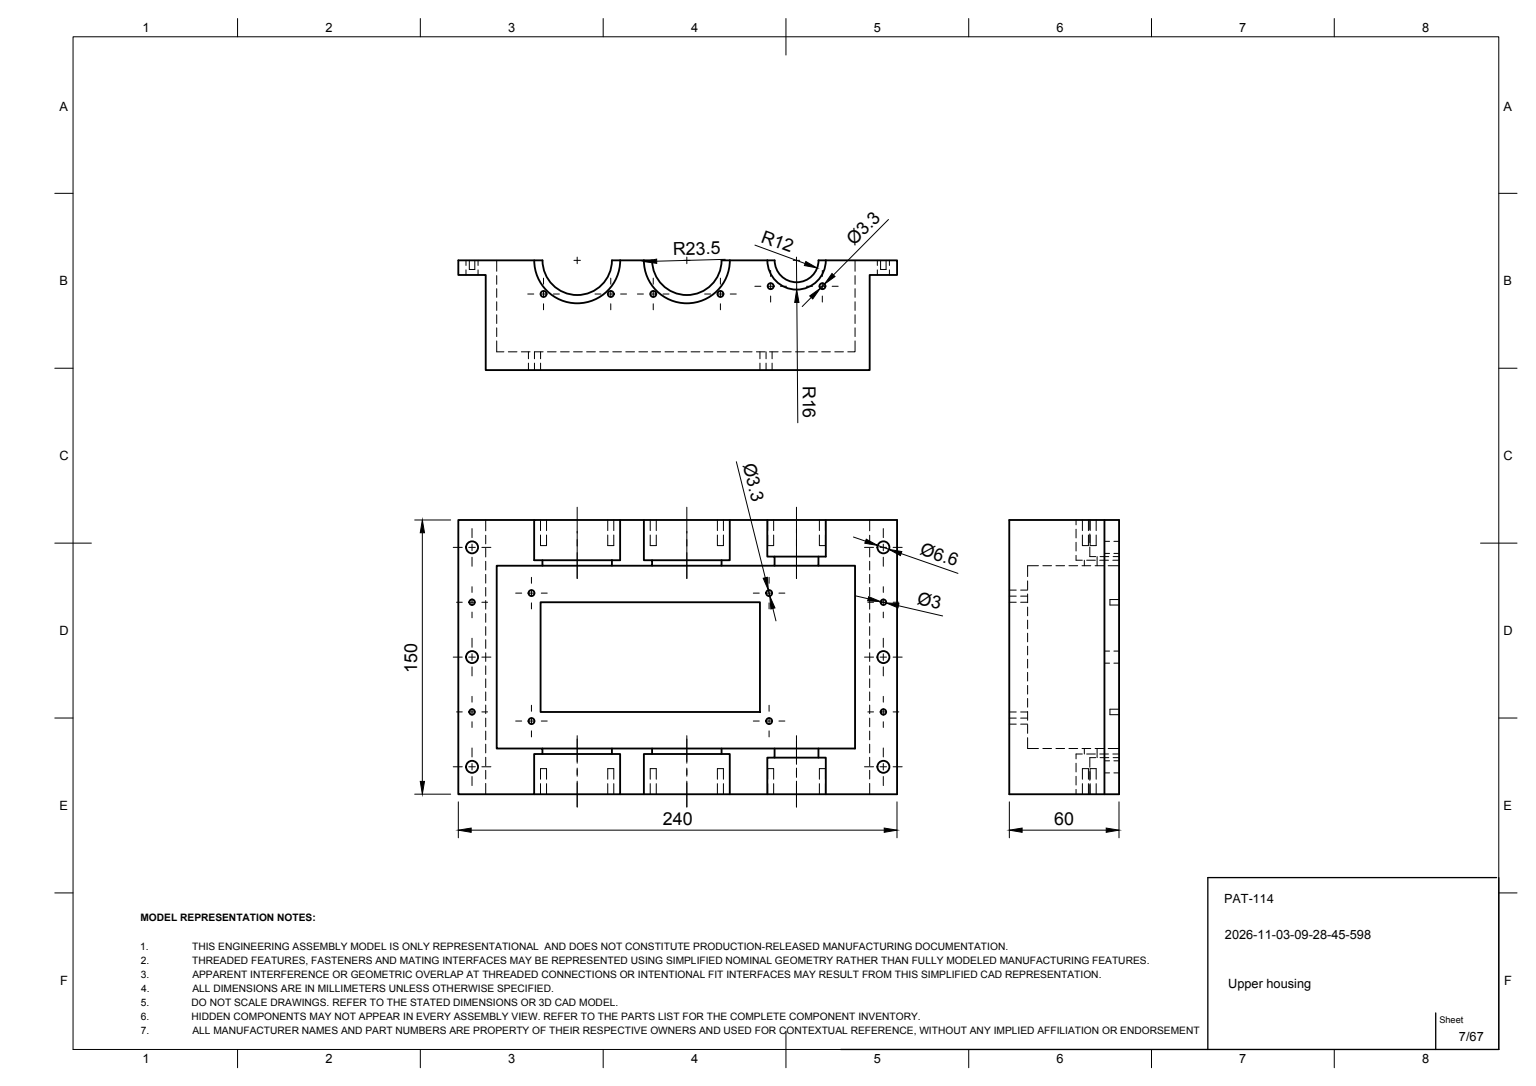
ISO-10303-21;
HEADER;
/* Generated by software containing ST-Developer
 * from STEP Tools, Inc. (www.steptools.com) 
 */

FILE_DESCRIPTION(
/* description */ ('Two-stage gear reducer in split housing'),
/* implementation_level */ '2;1');

FILE_NAME(
/* name */ 'Upper housing.step',
/* time_stamp */ '2026-10-28T03:22:31-07:00',
/* author */ (''),
/* organization */ (''),
/* preprocessor_version */ 'ST-DEVELOPER v20.2',
/* originating_system */ 'Autodesk Translation Framework v15.17.0.0',
/* authorisation */ '');

FILE_SCHEMA (('AUTOMOTIVE_DESIGN { 1 0 10303 214 3 1 1 }'));
ENDSEC;

DATA;
#10=MECHANICAL_DESIGN_GEOMETRIC_PRESENTATION_REPRESENTATION('',(#1236),#73366);
#1124=SHAPE_REPRESENTATION_RELATIONSHIP('SRR','None',#73611,#1180);
#1180=ADVANCED_BREP_SHAPE_REPRESENTATION('',(#1307),#73307);
#1236=STYLED_ITEM('',(#73967),#1307);
#1307=MANIFOLD_SOLID_BREP('Body1',#16124);
#1422=FACE_BOUND('',#3081,.T.);
#1423=FACE_BOUND('',#3082,.T.);
#1424=FACE_BOUND('',#3083,.T.);
#1425=FACE_BOUND('',#3084,.T.);
#1426=FACE_BOUND('',#3085,.T.);
#1427=FACE_BOUND('',#3089,.T.);
#1428=FACE_BOUND('',#3090,.T.);
#1429=FACE_BOUND('',#3091,.T.);
#1430=FACE_BOUND('',#3092,.T.);
#1431=FACE_BOUND('',#3093,.T.);
#1432=FACE_BOUND('',#3094,.T.);
#1433=FACE_BOUND('',#3097,.T.);
#1434=FACE_BOUND('',#3098,.T.);
#1435=FACE_BOUND('',#3099,.T.);
#1436=FACE_BOUND('',#3100,.T.);
#1437=FACE_BOUND('',#3101,.T.);
#1438=FACE_BOUND('',#3102,.T.);
#1439=FACE_BOUND('',#3138,.T.);
#1440=FACE_BOUND('',#3139,.T.);
#1441=FACE_BOUND('',#3140,.T.);
#1442=FACE_BOUND('',#3141,.T.);
#1443=FACE_BOUND('',#3142,.T.);
#1444=FACE_BOUND('',#3159,.T.);
#1445=FACE_BOUND('',#3160,.T.);
#1446=FACE_BOUND('',#3161,.T.);
#1447=FACE_BOUND('',#3164,.T.);
#1448=FACE_BOUND('',#3165,.T.);
#1449=FACE_BOUND('',#3166,.T.);
#1450=FACE_BOUND('',#3171,.T.);
#1451=FACE_BOUND('',#3172,.T.);
#1452=FACE_BOUND('',#3173,.T.);
#1453=FACE_BOUND('',#3174,.T.);
#1454=FACE_BOUND('',#3175,.T.);
#1455=FACE_BOUND('',#3178,.T.);
#1456=FACE_BOUND('',#3179,.T.);
#1457=FACE_BOUND('',#3180,.T.);
#1458=FACE_BOUND('',#3181,.T.);
#1459=FACE_BOUND('',#3182,.T.);
#1654=PLANE('',#17019);
#1655=PLANE('',#17020);
#1656=PLANE('',#17021);
#1657=PLANE('',#17022);
#1658=PLANE('',#17026);
#1659=PLANE('',#17030);
#1660=PLANE('',#17034);
#1661=PLANE('',#17038);
#1662=PLANE('',#17039);
#1663=PLANE('',#17046);
#1664=PLANE('',#17055);
#1665=PLANE('',#17057);
#1666=PLANE('',#17066);
#1667=PLANE('',#17073);
#1668=PLANE('',#17076);
#1669=PLANE('',#17077);
#1670=PLANE('',#17080);
#1671=PLANE('',#17083);
#1672=PLANE('',#17086);
#1673=PLANE('',#17089);
#1674=PLANE('',#17090);
#1675=PLANE('',#17098);
#1676=PLANE('',#17101);
#1677=PLANE('',#17102);
#1678=PLANE('',#17105);
#1679=PLANE('',#17108);
#1680=PLANE('',#17111);
#1681=PLANE('',#17114);
#1682=PLANE('',#17117);
#1683=PLANE('',#17121);
#1684=PLANE('',#17126);
#1685=PLANE('',#17127);
#1686=PLANE('',#17135);
#1687=PLANE('',#17138);
#1688=PLANE('',#17141);
#1689=PLANE('',#17144);
#1690=PLANE('',#17157);
#1691=PLANE('',#17158);
#1692=PLANE('',#17159);
#1693=PLANE('',#17160);
#1694=PLANE('',#17161);
#1695=PLANE('',#17162);
#1696=PLANE('',#17163);
#1697=PLANE('',#17164);
#1698=PLANE('',#17165);
#1699=PLANE('',#17166);
#2100=FACE_OUTER_BOUND('',#3061,.T.);
#2101=FACE_OUTER_BOUND('',#3062,.T.);
#2102=FACE_OUTER_BOUND('',#3063,.T.);
#2103=FACE_OUTER_BOUND('',#3064,.T.);
#2104=FACE_OUTER_BOUND('',#3065,.T.);
#2105=FACE_OUTER_BOUND('',#3066,.T.);
#2106=FACE_OUTER_BOUND('',#3067,.T.);
#2107=FACE_OUTER_BOUND('',#3068,.T.);
#2108=FACE_OUTER_BOUND('',#3069,.T.);
#2109=FACE_OUTER_BOUND('',#3070,.T.);
#2110=FACE_OUTER_BOUND('',#3071,.T.);
#2111=FACE_OUTER_BOUND('',#3072,.T.);
#2112=FACE_OUTER_BOUND('',#3073,.T.);
#2113=FACE_OUTER_BOUND('',#3074,.T.);
#2114=FACE_OUTER_BOUND('',#3075,.T.);
#2115=FACE_OUTER_BOUND('',#3076,.T.);
#2116=FACE_OUTER_BOUND('',#3077,.T.);
#2117=FACE_OUTER_BOUND('',#3078,.T.);
#2118=FACE_OUTER_BOUND('',#3079,.T.);
#2119=FACE_OUTER_BOUND('',#3080,.T.);
#2120=FACE_OUTER_BOUND('',#3086,.T.);
#2121=FACE_OUTER_BOUND('',#3087,.T.);
#2122=FACE_OUTER_BOUND('',#3088,.T.);
#2123=FACE_OUTER_BOUND('',#3095,.T.);
#2124=FACE_OUTER_BOUND('',#3096,.T.);
#2125=FACE_OUTER_BOUND('',#3103,.T.);
#2126=FACE_OUTER_BOUND('',#3104,.T.);
#2127=FACE_OUTER_BOUND('',#3105,.T.);
#2128=FACE_OUTER_BOUND('',#3106,.T.);
#2129=FACE_OUTER_BOUND('',#3107,.T.);
#2130=FACE_OUTER_BOUND('',#3108,.T.);
#2131=FACE_OUTER_BOUND('',#3109,.T.);
#2132=FACE_OUTER_BOUND('',#3110,.T.);
#2133=FACE_OUTER_BOUND('',#3111,.T.);
#2134=FACE_OUTER_BOUND('',#3112,.T.);
#2135=FACE_OUTER_BOUND('',#3113,.T.);
#2136=FACE_OUTER_BOUND('',#3114,.T.);
#2137=FACE_OUTER_BOUND('',#3115,.T.);
#2138=FACE_OUTER_BOUND('',#3116,.T.);
#2139=FACE_OUTER_BOUND('',#3117,.T.);
#2140=FACE_OUTER_BOUND('',#3118,.T.);
#2141=FACE_OUTER_BOUND('',#3119,.T.);
#2142=FACE_OUTER_BOUND('',#3120,.T.);
#2143=FACE_OUTER_BOUND('',#3121,.T.);
#2144=FACE_OUTER_BOUND('',#3122,.T.);
#2145=FACE_OUTER_BOUND('',#3123,.T.);
#2146=FACE_OUTER_BOUND('',#3124,.T.);
#2147=FACE_OUTER_BOUND('',#3125,.T.);
#2148=FACE_OUTER_BOUND('',#3126,.T.);
#2149=FACE_OUTER_BOUND('',#3127,.T.);
#2150=FACE_OUTER_BOUND('',#3128,.T.);
#2151=FACE_OUTER_BOUND('',#3129,.T.);
#2152=FACE_OUTER_BOUND('',#3130,.T.);
#2153=FACE_OUTER_BOUND('',#3131,.T.);
#2154=FACE_OUTER_BOUND('',#3132,.T.);
#2155=FACE_OUTER_BOUND('',#3133,.T.);
#2156=FACE_OUTER_BOUND('',#3134,.T.);
#2157=FACE_OUTER_BOUND('',#3135,.T.);
#2158=FACE_OUTER_BOUND('',#3136,.T.);
#2159=FACE_OUTER_BOUND('',#3137,.T.);
#2160=FACE_OUTER_BOUND('',#3143,.T.);
#2161=FACE_OUTER_BOUND('',#3144,.T.);
#2162=FACE_OUTER_BOUND('',#3145,.T.);
#2163=FACE_OUTER_BOUND('',#3146,.T.);
#2164=FACE_OUTER_BOUND('',#3147,.T.);
#2165=FACE_OUTER_BOUND('',#3148,.T.);
#2166=FACE_OUTER_BOUND('',#3149,.T.);
#2167=FACE_OUTER_BOUND('',#3150,.T.);
#2168=FACE_OUTER_BOUND('',#3151,.T.);
#2169=FACE_OUTER_BOUND('',#3152,.T.);
#2170=FACE_OUTER_BOUND('',#3153,.T.);
#2171=FACE_OUTER_BOUND('',#3154,.T.);
#2172=FACE_OUTER_BOUND('',#3155,.T.);
#2173=FACE_OUTER_BOUND('',#3156,.T.);
#2174=FACE_OUTER_BOUND('',#3157,.T.);
#2175=FACE_OUTER_BOUND('',#3158,.T.);
#2176=FACE_OUTER_BOUND('',#3162,.T.);
#2177=FACE_OUTER_BOUND('',#3163,.T.);
#2178=FACE_OUTER_BOUND('',#3167,.T.);
#2179=FACE_OUTER_BOUND('',#3168,.T.);
#2180=FACE_OUTER_BOUND('',#3169,.T.);
#2181=FACE_OUTER_BOUND('',#3170,.T.);
#2182=FACE_OUTER_BOUND('',#3176,.T.);
#2183=FACE_OUTER_BOUND('',#3177,.T.);
#3061=EDGE_LOOP('',(#10951,#10952,#10953,#10954));
#3062=EDGE_LOOP('',(#10955,#10956,#10957,#10958));
#3063=EDGE_LOOP('',(#10959,#10960,#10961,#10962));
#3064=EDGE_LOOP('',(#10963,#10964,#10965,#10966));
#3065=EDGE_LOOP('',(#10967,#10968,#10969,#10970));
#3066=EDGE_LOOP('',(#10971,#10972,#10973,#10974));
#3067=EDGE_LOOP('',(#10975,#10976,#10977,#10978));
#3068=EDGE_LOOP('',(#10979,#10980,#10981,#10982));
#3069=EDGE_LOOP('',(#10983,#10984,#10985,#10986));
#3070=EDGE_LOOP('',(#10987));
#3071=EDGE_LOOP('',(#10988,#10989,#10990,#10991));
#3072=EDGE_LOOP('',(#10992));
#3073=EDGE_LOOP('',(#10993,#10994,#10995,#10996));
#3074=EDGE_LOOP('',(#10997));
#3075=EDGE_LOOP('',(#10998,#10999,#11000,#11001));
#3076=EDGE_LOOP('',(#11002));
#3077=EDGE_LOOP('',(#11003,#11004,#11005,#11006));
#3078=EDGE_LOOP('',(#11007,#11008,#11009,#11010));
#3079=EDGE_LOOP('',(#11011,#11012,#11013,#11014));
#3080=EDGE_LOOP('',(#11015,#11016,#11017,#11018,#11019,#11020,#11021,#11022,
#11023,#11024,#11025,#11026));
#3081=EDGE_LOOP('',(#11027));
#3082=EDGE_LOOP('',(#11028));
#3083=EDGE_LOOP('',(#11029));
#3084=EDGE_LOOP('',(#11030));
#3085=EDGE_LOOP('',(#11031));
#3086=EDGE_LOOP('',(#11032,#11033,#11034,#11035));
#3087=EDGE_LOOP('',(#11036,#11037,#11038,#11039));
#3088=EDGE_LOOP('',(#11040,#11041,#11042,#11043,#11044,#11045,#11046,#11047,
#11048,#11049,#11050,#11051,#11052,#11053));
#3089=EDGE_LOOP('',(#11054));
#3090=EDGE_LOOP('',(#11055));
#3091=EDGE_LOOP('',(#11056));
#3092=EDGE_LOOP('',(#11057));
#3093=EDGE_LOOP('',(#11058));
#3094=EDGE_LOOP('',(#11059));
#3095=EDGE_LOOP('',(#11060,#11061,#11062,#11063));
#3096=EDGE_LOOP('',(#11064,#11065,#11066,#11067,#11068,#11069,#11070,#11071,
#11072,#11073,#11074,#11075,#11076,#11077));
#3097=EDGE_LOOP('',(#11078));
#3098=EDGE_LOOP('',(#11079));
#3099=EDGE_LOOP('',(#11080));
#3100=EDGE_LOOP('',(#11081));
#3101=EDGE_LOOP('',(#11082));
#3102=EDGE_LOOP('',(#11083));
#3103=EDGE_LOOP('',(#11084,#11085,#11086,#11087,#11088,#11089,#11090,#11091,
#11092,#11093));
#3104=EDGE_LOOP('',(#11094,#11095,#11096,#11097,#11098,#11099,#11100,#11101));
#3105=EDGE_LOOP('',(#11102,#11103,#11104,#11105,#11106,#11107,#11108,#11109));
#3106=EDGE_LOOP('',(#11110,#11111,#11112,#11113));
#3107=EDGE_LOOP('',(#11114));
#3108=EDGE_LOOP('',(#11115,#11116,#11117,#11118));
#3109=EDGE_LOOP('',(#11119));
#3110=EDGE_LOOP('',(#11120,#11121,#11122,#11123));
#3111=EDGE_LOOP('',(#11124));
#3112=EDGE_LOOP('',(#11125,#11126,#11127,#11128));
#3113=EDGE_LOOP('',(#11129));
#3114=EDGE_LOOP('',(#11130,#11131,#11132,#11133));
#3115=EDGE_LOOP('',(#11134,#11135,#11136,#11137));
#3116=EDGE_LOOP('',(#11138,#11139,#11140,#11141));
#3117=EDGE_LOOP('',(#11142,#11143,#11144,#11145));
#3118=EDGE_LOOP('',(#11146,#11147,#11148,#11149));
#3119=EDGE_LOOP('',(#11150,#11151,#11152,#11153));
#3120=EDGE_LOOP('',(#11154,#11155,#11156,#11157,#11158,#11159,#11160,#11161));
#3121=EDGE_LOOP('',(#11162,#11163,#11164,#11165,#11166,#11167,#11168,#11169));
#3122=EDGE_LOOP('',(#11170,#11171,#11172,#11173));
#3123=EDGE_LOOP('',(#11174));
#3124=EDGE_LOOP('',(#11175,#11176,#11177,#11178));
#3125=EDGE_LOOP('',(#11179));
#3126=EDGE_LOOP('',(#11180,#11181,#11182,#11183));
#3127=EDGE_LOOP('',(#11184));
#3128=EDGE_LOOP('',(#11185,#11186,#11187,#11188));
#3129=EDGE_LOOP('',(#11189));
#3130=EDGE_LOOP('',(#11190,#11191,#11192,#11193));
#3131=EDGE_LOOP('',(#11194,#11195,#11196,#11197));
#3132=EDGE_LOOP('',(#11198,#11199,#11200,#11201));
#3133=EDGE_LOOP('',(#11202,#11203,#11204,#11205));
#3134=EDGE_LOOP('',(#11206,#11207,#11208,#11209));
#3135=EDGE_LOOP('',(#11210,#11211,#11212,#11213));
#3136=EDGE_LOOP('',(#11214,#11215,#11216,#11217,#11218,#11219,#11220,#11221,
#11222,#11223));
#3137=EDGE_LOOP('',(#11224,#11225,#11226,#11227,#11228,#11229,#11230,#11231,
#11232,#11233,#11234,#11235));
#3138=EDGE_LOOP('',(#11236));
#3139=EDGE_LOOP('',(#11237));
#3140=EDGE_LOOP('',(#11238));
#3141=EDGE_LOOP('',(#11239));
#3142=EDGE_LOOP('',(#11240));
#3143=EDGE_LOOP('',(#11241,#11242,#11243,#11244));
#3144=EDGE_LOOP('',(#11245));
#3145=EDGE_LOOP('',(#11246,#11247,#11248,#11249));
#3146=EDGE_LOOP('',(#11250));
#3147=EDGE_LOOP('',(#11251,#11252,#11253,#11254));
#3148=EDGE_LOOP('',(#11255));
#3149=EDGE_LOOP('',(#11256,#11257,#11258,#11259));
#3150=EDGE_LOOP('',(#11260));
#3151=EDGE_LOOP('',(#11261,#11262,#11263,#11264));
#3152=EDGE_LOOP('',(#11265,#11266,#11267,#11268));
#3153=EDGE_LOOP('',(#11269,#11270,#11271,#11272));
#3154=EDGE_LOOP('',(#11273,#11274,#11275,#11276));
#3155=EDGE_LOOP('',(#11277,#11278,#11279,#11280));
#3156=EDGE_LOOP('',(#11281,#11282,#11283,#11284));
#3157=EDGE_LOOP('',(#11285,#11286,#11287,#11288));
#3158=EDGE_LOOP('',(#11289,#11290,#11291,#11292));
#3159=EDGE_LOOP('',(#11293));
#3160=EDGE_LOOP('',(#11294));
#3161=EDGE_LOOP('',(#11295));
#3162=EDGE_LOOP('',(#11296,#11297,#11298,#11299));
#3163=EDGE_LOOP('',(#11300,#11301,#11302,#11303));
#3164=EDGE_LOOP('',(#11304));
#3165=EDGE_LOOP('',(#11305));
#3166=EDGE_LOOP('',(#11306));
#3167=EDGE_LOOP('',(#11307,#11308,#11309,#11310));
#3168=EDGE_LOOP('',(#11311,#11312,#11313,#11314));
#3169=EDGE_LOOP('',(#11315,#11316,#11317,#11318));
#3170=EDGE_LOOP('',(#11319,#11320,#11321,#11322));
#3171=EDGE_LOOP('',(#11323,#11324,#11325,#11326));
#3172=EDGE_LOOP('',(#11327));
#3173=EDGE_LOOP('',(#11328));
#3174=EDGE_LOOP('',(#11329));
#3175=EDGE_LOOP('',(#11330));
#3176=EDGE_LOOP('',(#11331,#11332,#11333,#11334));
#3177=EDGE_LOOP('',(#11335,#11336,#11337,#11338));
#3178=EDGE_LOOP('',(#11339,#11340,#11341,#11342));
#3179=EDGE_LOOP('',(#11343));
#3180=EDGE_LOOP('',(#11344));
#3181=EDGE_LOOP('',(#11345));
#3182=EDGE_LOOP('',(#11346));
#4186=LINE('',#23251,#5210);
#4187=LINE('',#23257,#5211);
#4188=LINE('',#23263,#5212);
#4189=LINE('',#23269,#5213);
#4190=LINE('',#23274,#5214);
#4191=LINE('',#23276,#5215);
#4192=LINE('',#23278,#5216);
#4193=LINE('',#23279,#5217);
#4194=LINE('',#23282,#5218);
#4195=LINE('',#23284,#5219);
#4196=LINE('',#23285,#5220);
#4197=LINE('',#23288,#5221);
#4198=LINE('',#23290,#5222);
#4199=LINE('',#23291,#5223);
#4200=LINE('',#23293,#5224);
#4201=LINE('',#23294,#5225);
#4202=LINE('',#23299,#5226);
#4203=LINE('',#23306,#5227);
#4204=LINE('',#23313,#5228);
#4205=LINE('',#23320,#5229);
#4206=LINE('',#23326,#5230);
#4207=LINE('',#23330,#5231);
#4208=LINE('',#23334,#5232);
#4209=LINE('',#23337,#5233);
#4210=LINE('',#23340,#5234);
#4211=LINE('',#23343,#5235);
#4212=LINE('',#23346,#5236);
#4213=LINE('',#23348,#5237);
#4214=LINE('',#23350,#5238);
#4215=LINE('',#23352,#5239);
#4216=LINE('',#23354,#5240);
#4217=LINE('',#23356,#5241);
#4218=LINE('',#23358,#5242);
#4219=LINE('',#23360,#5243);
#4220=LINE('',#23361,#5244);
#4221=LINE('',#23375,#5245);
#4222=LINE('',#23380,#5246);
#4223=LINE('',#23384,#5247);
#4224=LINE('',#23386,#5248);
#4225=LINE('',#23388,#5249);
#4226=LINE('',#23390,#5250);
#4227=LINE('',#23392,#5251);
#4228=LINE('',#23394,#5252);
#4229=LINE('',#23396,#5253);
#4230=LINE('',#23398,#5254);
#4231=LINE('',#23402,#5255);
#4232=LINE('',#23405,#5256);
#4233=LINE('',#23416,#5257);
#4234=LINE('',#23420,#5258);
#4235=LINE('',#23424,#5259);
#4236=LINE('',#23428,#5260);
#4237=LINE('',#23430,#5261);
#4238=LINE('',#23432,#5262);
#4239=LINE('',#23434,#5263);
#4240=LINE('',#23436,#5264);
#4241=LINE('',#23438,#5265);
#4242=LINE('',#23440,#5266);
#4243=LINE('',#23441,#5267);
#4244=LINE('',#23452,#5268);
#4245=LINE('',#23456,#5269);
#4246=LINE('',#23460,#5270);
#4247=LINE('',#23462,#5271);
#4248=LINE('',#23464,#5272);
#4249=LINE('',#23465,#5273);
#4250=LINE('',#23468,#5274);
#4251=LINE('',#23470,#5275);
#4252=LINE('',#23471,#5276);
#4253=LINE('',#23474,#5277);
#4254=LINE('',#23476,#5278);
#4255=LINE('',#23478,#5279);
#4256=LINE('',#23479,#5280);
#4257=LINE('',#23483,#5281);
#4258=LINE('',#23488,#5282);
#4259=LINE('',#23492,#5283);
#4260=LINE('',#23497,#5284);
#4261=LINE('',#23503,#5285);
#4262=LINE('',#23507,#5286);
#4263=LINE('',#23511,#5287);
#4264=LINE('',#23514,#5288);
#4265=LINE('',#23518,#5289);
#4266=LINE('',#23521,#5290);
#4267=LINE('',#23524,#5291);
#4268=LINE('',#23526,#5292);
#4269=LINE('',#23527,#5293);
#4270=LINE('',#23530,#5294);
#4271=LINE('',#23532,#5295);
#4272=LINE('',#23534,#5296);
#4273=LINE('',#23535,#5297);
#4274=LINE('',#23539,#5298);
#4275=LINE('',#23544,#5299);
#4276=LINE('',#23548,#5300);
#4277=LINE('',#23553,#5301);
#4278=LINE('',#23559,#5302);
#4279=LINE('',#23563,#5303);
#4280=LINE('',#23566,#5304);
#4281=LINE('',#23570,#5305);
#4282=LINE('',#23573,#5306);
#4283=LINE('',#23577,#5307);
#4284=LINE('',#23580,#5308);
#4285=LINE('',#23582,#5309);
#4286=LINE('',#23584,#5310);
#4287=LINE('',#23585,#5311);
#4288=LINE('',#23587,#5312);
#4289=LINE('',#23588,#5313);
#4290=LINE('',#23601,#5314);
#4291=LINE('',#23606,#5315);
#4292=LINE('',#23611,#5316);
#4293=LINE('',#23616,#5317);
#4294=LINE('',#23621,#5318);
#4295=LINE('',#23625,#5319);
#4296=LINE('',#23629,#5320);
#4297=LINE('',#23633,#5321);
#4298=LINE('',#23637,#5322);
#4299=LINE('',#23641,#5323);
#4300=LINE('',#23644,#5324);
#4301=LINE('',#23646,#5325);
#4302=LINE('',#23648,#5326);
#4303=LINE('',#23650,#5327);
#4304=LINE('',#23652,#5328);
#4305=LINE('',#23654,#5329);
#4306=LINE('',#23656,#5330);
#4307=LINE('',#23659,#5331);
#5210=VECTOR('',#18982,0.164999999999999);
#5211=VECTOR('',#18989,0.165);
#5212=VECTOR('',#18996,0.165);
#5213=VECTOR('',#19003,0.164999999999999);
#5214=VECTOR('',#19008,1.);
#5215=VECTOR('',#19009,1.);
#5216=VECTOR('',#19010,1.);
#5217=VECTOR('',#19011,1.);
#5218=VECTOR('',#19014,1.);
#5219=VECTOR('',#19015,1.);
#5220=VECTOR('',#19016,1.);
#5221=VECTOR('',#19019,1.);
#5222=VECTOR('',#19020,1.);
#5223=VECTOR('',#19021,1.);
#5224=VECTOR('',#19024,1.);
#5225=VECTOR('',#19025,1.);
#5226=VECTOR('',#19030,0.164999999999999);
#5227=VECTOR('',#19039,0.164999999999999);
#5228=VECTOR('',#19048,0.164999999999999);
#5229=VECTOR('',#19057,0.164999999999999);
#5230=VECTOR('',#19064,1.);
#5231=VECTOR('',#19067,1.);
#5232=VECTOR('',#19072,1.);
#5233=VECTOR('',#19075,1.);
#5234=VECTOR('',#19078,1.);
#5235=VECTOR('',#19081,1.);
#5236=VECTOR('',#19084,1.);
#5237=VECTOR('',#19085,1.);
#5238=VECTOR('',#19086,1.);
#5239=VECTOR('',#19087,1.);
#5240=VECTOR('',#19088,1.);
#5241=VECTOR('',#19089,1.);
#5242=VECTOR('',#19090,1.);
#5243=VECTOR('',#19091,1.);
#5244=VECTOR('',#19092,1.);
#5245=VECTOR('',#19105,1.);
#5246=VECTOR('',#19112,1.);
#5247=VECTOR('',#19117,1.);
#5248=VECTOR('',#19118,1.);
#5249=VECTOR('',#19119,1.);
#5250=VECTOR('',#19120,1.);
#5251=VECTOR('',#19121,1.);
#5252=VECTOR('',#19122,1.);
#5253=VECTOR('',#19123,1.);
#5254=VECTOR('',#19124,1.);
#5255=VECTOR('',#19127,1.);
#5256=VECTOR('',#19130,1.);
#5257=VECTOR('',#19141,1.);
#5258=VECTOR('',#19146,1.);
#5259=VECTOR('',#19149,1.);
#5260=VECTOR('',#19152,1.);
#5261=VECTOR('',#19153,1.);
#5262=VECTOR('',#19154,1.);
#5263=VECTOR('',#19155,1.);
#5264=VECTOR('',#19156,1.);
#5265=VECTOR('',#19157,1.);
#5266=VECTOR('',#19158,1.);
#5267=VECTOR('',#19159,1.);
#5268=VECTOR('',#19170,1.);
#5269=VECTOR('',#19173,1.);
#5270=VECTOR('',#19176,1.);
#5271=VECTOR('',#19177,1.);
#5272=VECTOR('',#19178,1.);
#5273=VECTOR('',#19179,1.);
#5274=VECTOR('',#19182,1.);
#5275=VECTOR('',#19183,1.);
#5276=VECTOR('',#19184,1.);
#5277=VECTOR('',#19187,1.);
#5278=VECTOR('',#19188,1.);
#5279=VECTOR('',#19189,1.);
#5280=VECTOR('',#19190,1.);
#5281=VECTOR('',#19195,0.165);
#5282=VECTOR('',#19202,0.165);
#5283=VECTOR('',#19207,0.165);
#5284=VECTOR('',#19214,0.165);
#5285=VECTOR('',#19221,1.);
#5286=VECTOR('',#19228,1.);
#5287=VECTOR('',#19233,1.);
#5288=VECTOR('',#19236,1.);
#5289=VECTOR('',#19241,1.);
#5290=VECTOR('',#19246,1.);
#5291=VECTOR('',#19249,1.);
#5292=VECTOR('',#19250,1.);
#5293=VECTOR('',#19251,1.);
#5294=VECTOR('',#19254,1.);
#5295=VECTOR('',#19255,1.);
#5296=VECTOR('',#19256,1.);
#5297=VECTOR('',#19257,1.);
#5298=VECTOR('',#19262,0.165);
#5299=VECTOR('',#19269,0.165);
#5300=VECTOR('',#19274,0.165);
#5301=VECTOR('',#19281,0.165);
#5302=VECTOR('',#19290,1.);
#5303=VECTOR('',#19295,1.);
#5304=VECTOR('',#19298,1.);
#5305=VECTOR('',#19303,1.);
#5306=VECTOR('',#19308,1.);
#5307=VECTOR('',#19313,1.);
#5308=VECTOR('',#19316,1.);
#5309=VECTOR('',#19317,1.);
#5310=VECTOR('',#19318,1.);
#5311=VECTOR('',#19319,1.);
#5312=VECTOR('',#19322,1.);
#5313=VECTOR('',#19323,1.);
#5314=VECTOR('',#19336,0.149999999999999);
#5315=VECTOR('',#19343,0.149999999999999);
#5316=VECTOR('',#19350,0.15);
#5317=VECTOR('',#19357,0.15);
#5318=VECTOR('',#19364,0.329999999999998);
#5319=VECTOR('',#19369,0.33);
#5320=VECTOR('',#19374,0.33);
#5321=VECTOR('',#19379,0.33);
#5322=VECTOR('',#19384,0.329999999999998);
#5323=VECTOR('',#19389,0.329999999999998);
#5324=VECTOR('',#19394,1.);
#5325=VECTOR('',#19397,1.);
#5326=VECTOR('',#19400,1.);
#5327=VECTOR('',#19403,1.);
#5328=VECTOR('',#19406,1.);
#5329=VECTOR('',#19409,1.);
#5330=VECTOR('',#19412,1.);
#5331=VECTOR('',#19417,1.);
#6196=CIRCLE('',#17008,0.164999999999999);
#6197=CIRCLE('',#17009,0.164999999999999);
#6198=CIRCLE('',#17011,0.165);
#6199=CIRCLE('',#17012,0.165);
#6200=CIRCLE('',#17014,0.165);
#6201=CIRCLE('',#17015,0.165);
#6202=CIRCLE('',#17017,0.164999999999999);
#6203=CIRCLE('',#17018,0.164999999999999);
#6204=CIRCLE('',#17024,0.164999999999999);
#6205=CIRCLE('',#17025,0.164999999999999);
#6206=CIRCLE('',#17028,0.164999999999999);
#6207=CIRCLE('',#17029,0.164999999999999);
#6208=CIRCLE('',#17032,0.164999999999999);
#6209=CIRCLE('',#17033,0.164999999999999);
#6210=CIRCLE('',#17036,0.164999999999999);
#6211=CIRCLE('',#17037,0.164999999999999);
#6212=CIRCLE('',#17040,2.35);
#6213=CIRCLE('',#17041,1.9);
#6214=CIRCLE('',#17043,2.35);
#6215=CIRCLE('',#17045,1.9);
#6216=CIRCLE('',#17047,0.149999999999999);
#6217=CIRCLE('',#17048,0.329999999999998);
#6218=CIRCLE('',#17049,0.329999999999998);
#6219=CIRCLE('',#17050,0.329999999999998);
#6220=CIRCLE('',#17051,0.149999999999999);
#6221=CIRCLE('',#17053,2.35);
#6222=CIRCLE('',#17054,2.35);
#6223=CIRCLE('',#17056,1.9);
#6224=CIRCLE('',#17058,1.6);
#6225=CIRCLE('',#17059,2.35);
#6226=CIRCLE('',#17060,0.165);
#6227=CIRCLE('',#17061,0.165);
#6228=CIRCLE('',#17062,0.165);
#6229=CIRCLE('',#17063,0.165);
#6230=CIRCLE('',#17065,1.9);
#6231=CIRCLE('',#17067,2.35);
#6232=CIRCLE('',#17068,1.6);
#6233=CIRCLE('',#17069,0.165);
#6234=CIRCLE('',#17070,0.165);
#6235=CIRCLE('',#17071,0.165);
#6236=CIRCLE('',#17072,0.165);
#6237=CIRCLE('',#17074,1.9);
#6238=CIRCLE('',#17075,1.2);
#6239=CIRCLE('',#17079,0.165);
#6240=CIRCLE('',#17082,0.165);
#6241=CIRCLE('',#17085,0.165);
#6242=CIRCLE('',#17088,0.165);
#6243=CIRCLE('',#17091,2.35);
#6244=CIRCLE('',#17092,1.9);
#6245=CIRCLE('',#17095,1.9);
#6246=CIRCLE('',#17097,2.35);
#6247=CIRCLE('',#17099,1.9);
#6248=CIRCLE('',#17104,0.165);
#6249=CIRCLE('',#17107,0.165);
#6250=CIRCLE('',#17110,0.165);
#6251=CIRCLE('',#17113,0.165);
#6252=CIRCLE('',#17116,1.6);
#6253=CIRCLE('',#17118,1.2);
#6254=CIRCLE('',#17120,1.6);
#6255=CIRCLE('',#17122,1.2);
#6256=CIRCLE('',#17125,1.2);
#6257=CIRCLE('',#17128,0.15);
#6258=CIRCLE('',#17129,0.33);
#6259=CIRCLE('',#17130,0.33);
#6260=CIRCLE('',#17131,0.33);
#6261=CIRCLE('',#17132,0.15);
#6262=CIRCLE('',#17134,0.149999999999999);
#6263=CIRCLE('',#17137,0.149999999999999);
#6264=CIRCLE('',#17140,0.15);
#6265=CIRCLE('',#17143,0.15);
#6266=CIRCLE('',#17146,0.329999999999998);
#6267=CIRCLE('',#17148,0.33);
#6268=CIRCLE('',#17150,0.33);
#6269=CIRCLE('',#17152,0.33);
#6270=CIRCLE('',#17154,0.329999999999998);
#6271=CIRCLE('',#17156,0.329999999999998);
#6972=VERTEX_POINT('',#23248);
#6973=VERTEX_POINT('',#23250);
#6974=VERTEX_POINT('',#23254);
#6975=VERTEX_POINT('',#23256);
#6976=VERTEX_POINT('',#23260);
#6977=VERTEX_POINT('',#23262);
#6978=VERTEX_POINT('',#23266);
#6979=VERTEX_POINT('',#23268);
#6980=VERTEX_POINT('',#23272);
#6981=VERTEX_POINT('',#23273);
#6982=VERTEX_POINT('',#23275);
#6983=VERTEX_POINT('',#23277);
#6984=VERTEX_POINT('',#23281);
#6985=VERTEX_POINT('',#23283);
#6986=VERTEX_POINT('',#23287);
#6987=VERTEX_POINT('',#23289);
#6988=VERTEX_POINT('',#23296);
#6989=VERTEX_POINT('',#23298);
#6990=VERTEX_POINT('',#23303);
#6991=VERTEX_POINT('',#23305);
#6992=VERTEX_POINT('',#23310);
#6993=VERTEX_POINT('',#23312);
#6994=VERTEX_POINT('',#23317);
#6995=VERTEX_POINT('',#23319);
#6996=VERTEX_POINT('',#23324);
#6997=VERTEX_POINT('',#23325);
#6998=VERTEX_POINT('',#23327);
#6999=VERTEX_POINT('',#23329);
#7000=VERTEX_POINT('',#23333);
#7001=VERTEX_POINT('',#23335);
#7002=VERTEX_POINT('',#23339);
#7003=VERTEX_POINT('',#23341);
#7004=VERTEX_POINT('',#23345);
#7005=VERTEX_POINT('',#23347);
#7006=VERTEX_POINT('',#23349);
#7007=VERTEX_POINT('',#23351);
#7008=VERTEX_POINT('',#23353);
#7009=VERTEX_POINT('',#23355);
#7010=VERTEX_POINT('',#23357);
#7011=VERTEX_POINT('',#23359);
#7012=VERTEX_POINT('',#23362);
#7013=VERTEX_POINT('',#23364);
#7014=VERTEX_POINT('',#23366);
#7015=VERTEX_POINT('',#23368);
#7016=VERTEX_POINT('',#23370);
#7017=VERTEX_POINT('',#23373);
#7018=VERTEX_POINT('',#23374);
#7019=VERTEX_POINT('',#23379);
#7020=VERTEX_POINT('',#23383);
#7021=VERTEX_POINT('',#23385);
#7022=VERTEX_POINT('',#23387);
#7023=VERTEX_POINT('',#23389);
#7024=VERTEX_POINT('',#23391);
#7025=VERTEX_POINT('',#23393);
#7026=VERTEX_POINT('',#23395);
#7027=VERTEX_POINT('',#23397);
#7028=VERTEX_POINT('',#23399);
#7029=VERTEX_POINT('',#23401);
#7030=VERTEX_POINT('',#23403);
#7031=VERTEX_POINT('',#23406);
#7032=VERTEX_POINT('',#23408);
#7033=VERTEX_POINT('',#23410);
#7034=VERTEX_POINT('',#23412);
#7035=VERTEX_POINT('',#23415);
#7036=VERTEX_POINT('',#23419);
#7037=VERTEX_POINT('',#23421);
#7038=VERTEX_POINT('',#23423);
#7039=VERTEX_POINT('',#23425);
#7040=VERTEX_POINT('',#23427);
#7041=VERTEX_POINT('',#23429);
#7042=VERTEX_POINT('',#23431);
#7043=VERTEX_POINT('',#23433);
#7044=VERTEX_POINT('',#23435);
#7045=VERTEX_POINT('',#23437);
#7046=VERTEX_POINT('',#23439);
#7047=VERTEX_POINT('',#23442);
#7048=VERTEX_POINT('',#23444);
#7049=VERTEX_POINT('',#23446);
#7050=VERTEX_POINT('',#23448);
#7051=VERTEX_POINT('',#23451);
#7052=VERTEX_POINT('',#23453);
#7053=VERTEX_POINT('',#23455);
#7054=VERTEX_POINT('',#23457);
#7055=VERTEX_POINT('',#23459);
#7056=VERTEX_POINT('',#23461);
#7057=VERTEX_POINT('',#23463);
#7058=VERTEX_POINT('',#23467);
#7059=VERTEX_POINT('',#23469);
#7060=VERTEX_POINT('',#23473);
#7061=VERTEX_POINT('',#23475);
#7062=VERTEX_POINT('',#23477);
#7063=VERTEX_POINT('',#23481);
#7064=VERTEX_POINT('',#23486);
#7065=VERTEX_POINT('',#23491);
#7066=VERTEX_POINT('',#23496);
#7067=VERTEX_POINT('',#23501);
#7068=VERTEX_POINT('',#23502);
#7069=VERTEX_POINT('',#23509);
#7070=VERTEX_POINT('',#23513);
#7071=VERTEX_POINT('',#23517);
#7072=VERTEX_POINT('',#23523);
#7073=VERTEX_POINT('',#23525);
#7074=VERTEX_POINT('',#23529);
#7075=VERTEX_POINT('',#23531);
#7076=VERTEX_POINT('',#23533);
#7077=VERTEX_POINT('',#23537);
#7078=VERTEX_POINT('',#23542);
#7079=VERTEX_POINT('',#23547);
#7080=VERTEX_POINT('',#23552);
#7081=VERTEX_POINT('',#23557);
#7082=VERTEX_POINT('',#23561);
#7083=VERTEX_POINT('',#23565);
#7084=VERTEX_POINT('',#23569);
#7085=VERTEX_POINT('',#23575);
#7086=VERTEX_POINT('',#23579);
#7087=VERTEX_POINT('',#23581);
#7088=VERTEX_POINT('',#23583);
#7089=VERTEX_POINT('',#23589);
#7090=VERTEX_POINT('',#23591);
#7091=VERTEX_POINT('',#23593);
#7092=VERTEX_POINT('',#23595);
#7093=VERTEX_POINT('',#23597);
#7094=VERTEX_POINT('',#23600);
#7095=VERTEX_POINT('',#23605);
#7096=VERTEX_POINT('',#23610);
#7097=VERTEX_POINT('',#23615);
#7098=VERTEX_POINT('',#23620);
#7099=VERTEX_POINT('',#23624);
#7100=VERTEX_POINT('',#23628);
#7101=VERTEX_POINT('',#23632);
#7102=VERTEX_POINT('',#23636);
#7103=VERTEX_POINT('',#23640);
#8529=EDGE_CURVE('',#6972,#6972,#6196,.T.);
#8530=EDGE_CURVE('',#6972,#6973,#4186,.T.);
#8531=EDGE_CURVE('',#6973,#6973,#6197,.T.);
#8532=EDGE_CURVE('',#6974,#6974,#6198,.T.);
#8533=EDGE_CURVE('',#6974,#6975,#4187,.T.);
#8534=EDGE_CURVE('',#6975,#6975,#6199,.T.);
#8535=EDGE_CURVE('',#6976,#6976,#6200,.T.);
#8536=EDGE_CURVE('',#6976,#6977,#4188,.T.);
#8537=EDGE_CURVE('',#6977,#6977,#6201,.T.);
#8538=EDGE_CURVE('',#6978,#6978,#6202,.T.);
#8539=EDGE_CURVE('',#6978,#6979,#4189,.T.);
#8540=EDGE_CURVE('',#6979,#6979,#6203,.T.);
#8541=EDGE_CURVE('',#6980,#6981,#4190,.T.);
#8542=EDGE_CURVE('',#6980,#6982,#4191,.T.);
#8543=EDGE_CURVE('',#6983,#6982,#4192,.T.);
#8544=EDGE_CURVE('',#6981,#6983,#4193,.T.);
#8545=EDGE_CURVE('',#6981,#6984,#4194,.T.);
#8546=EDGE_CURVE('',#6985,#6983,#4195,.T.);
#8547=EDGE_CURVE('',#6984,#6985,#4196,.T.);
#8548=EDGE_CURVE('',#6984,#6986,#4197,.T.);
#8549=EDGE_CURVE('',#6987,#6985,#4198,.T.);
#8550=EDGE_CURVE('',#6986,#6987,#4199,.T.);
#8551=EDGE_CURVE('',#6986,#6980,#4200,.T.);
#8552=EDGE_CURVE('',#6982,#6987,#4201,.T.);
#8553=EDGE_CURVE('',#6988,#6988,#6204,.T.);
#8554=EDGE_CURVE('',#6988,#6989,#4202,.T.);
#8555=EDGE_CURVE('',#6989,#6989,#6205,.T.);
#8556=EDGE_CURVE('',#6990,#6990,#6206,.T.);
#8557=EDGE_CURVE('',#6990,#6991,#4203,.T.);
#8558=EDGE_CURVE('',#6991,#6991,#6207,.T.);
#8559=EDGE_CURVE('',#6992,#6992,#6208,.T.);
#8560=EDGE_CURVE('',#6992,#6993,#4204,.T.);
#8561=EDGE_CURVE('',#6993,#6993,#6209,.T.);
#8562=EDGE_CURVE('',#6994,#6994,#6210,.T.);
#8563=EDGE_CURVE('',#6994,#6995,#4205,.T.);
#8564=EDGE_CURVE('',#6995,#6995,#6211,.T.);
#8565=EDGE_CURVE('',#6996,#6997,#4206,.T.);
#8566=EDGE_CURVE('',#6996,#6998,#6212,.T.);
#8567=EDGE_CURVE('',#6999,#6998,#4207,.T.);
#8568=EDGE_CURVE('',#6997,#6999,#6213,.T.);
#8569=EDGE_CURVE('',#7000,#6996,#4208,.T.);
#8570=EDGE_CURVE('',#7001,#7000,#6214,.T.);
#8571=EDGE_CURVE('',#6998,#7001,#4209,.T.);
#8572=EDGE_CURVE('',#7002,#6999,#4210,.T.);
#8573=EDGE_CURVE('',#7003,#7002,#6215,.T.);
#8574=EDGE_CURVE('',#6997,#7003,#4211,.T.);
#8575=EDGE_CURVE('',#7004,#7001,#4212,.T.);
#8576=EDGE_CURVE('',#7005,#7004,#4213,.T.);
#8577=EDGE_CURVE('',#7006,#7005,#4214,.T.);
#8578=EDGE_CURVE('',#7006,#7007,#4215,.T.);
#8579=EDGE_CURVE('',#7007,#7008,#4216,.T.);
#8580=EDGE_CURVE('',#7008,#7009,#4217,.T.);
#8581=EDGE_CURVE('',#7009,#7010,#4218,.T.);
#8582=EDGE_CURVE('',#7010,#7011,#4219,.T.);
#8583=EDGE_CURVE('',#7011,#7002,#4220,.T.);
#8584=EDGE_CURVE('',#7012,#7012,#6216,.T.);
#8585=EDGE_CURVE('',#7013,#7013,#6217,.T.);
#8586=EDGE_CURVE('',#7014,#7014,#6218,.T.);
#8587=EDGE_CURVE('',#7015,#7015,#6219,.T.);
#8588=EDGE_CURVE('',#7016,#7016,#6220,.T.);
#8589=EDGE_CURVE('',#7017,#7018,#4221,.T.);
#8590=EDGE_CURVE('',#7017,#7007,#6221,.T.);
#8591=EDGE_CURVE('',#7018,#7006,#6222,.T.);
#8592=EDGE_CURVE('',#7019,#7017,#4222,.T.);
#8593=EDGE_CURVE('',#7008,#7019,#6223,.T.);
#8594=EDGE_CURVE('',#7005,#7020,#4223,.T.);
#8595=EDGE_CURVE('',#7021,#7020,#4224,.T.);
#8596=EDGE_CURVE('',#7021,#7022,#4225,.T.);
#8597=EDGE_CURVE('',#7023,#7022,#4226,.T.);
#8598=EDGE_CURVE('',#7024,#7023,#4227,.T.);
#8599=EDGE_CURVE('',#7025,#7024,#4228,.T.);
#8600=EDGE_CURVE('',#7026,#7025,#4229,.T.);
#8601=EDGE_CURVE('',#7026,#7027,#4230,.T.);
#8602=EDGE_CURVE('',#7027,#7028,#6224,.T.);
#8603=EDGE_CURVE('',#7028,#7029,#4231,.T.);
#8604=EDGE_CURVE('',#7029,#7030,#6225,.T.);
#8605=EDGE_CURVE('',#7030,#7018,#4232,.T.);
#8606=EDGE_CURVE('',#7031,#7031,#6226,.T.);
#8607=EDGE_CURVE('',#7032,#7032,#6227,.T.);
#8608=EDGE_CURVE('',#7033,#7033,#6228,.T.);
#8609=EDGE_CURVE('',#7034,#7034,#6229,.T.);
#8610=EDGE_CURVE('',#7035,#7019,#4233,.T.);
#8611=EDGE_CURVE('',#7009,#7035,#6230,.T.);
#8612=EDGE_CURVE('',#7000,#7036,#4234,.T.);
#8613=EDGE_CURVE('',#7036,#7037,#6231,.T.);
#8614=EDGE_CURVE('',#7037,#7038,#4235,.T.);
#8615=EDGE_CURVE('',#7038,#7039,#6232,.T.);
#8616=EDGE_CURVE('',#7039,#7040,#4236,.T.);
#8617=EDGE_CURVE('',#7040,#7041,#4237,.T.);
#8618=EDGE_CURVE('',#7042,#7041,#4238,.T.);
#8619=EDGE_CURVE('',#7042,#7043,#4239,.T.);
#8620=EDGE_CURVE('',#7044,#7043,#4240,.T.);
#8621=EDGE_CURVE('',#7045,#7044,#4241,.T.);
#8622=EDGE_CURVE('',#7046,#7045,#4242,.T.);
#8623=EDGE_CURVE('',#7004,#7046,#4243,.T.);
#8624=EDGE_CURVE('',#7047,#7047,#6233,.T.);
#8625=EDGE_CURVE('',#7048,#7048,#6234,.T.);
#8626=EDGE_CURVE('',#7049,#7049,#6235,.T.);
#8627=EDGE_CURVE('',#7050,#7050,#6236,.T.);
#8628=EDGE_CURVE('',#7051,#7035,#4244,.T.);
#8629=EDGE_CURVE('',#7051,#7052,#6237,.T.);
#8630=EDGE_CURVE('',#7053,#7052,#4245,.T.);
#8631=EDGE_CURVE('',#7053,#7054,#6238,.T.);
#8632=EDGE_CURVE('',#7055,#7054,#4246,.T.);
#8633=EDGE_CURVE('',#7055,#7056,#4247,.T.);
#8634=EDGE_CURVE('',#7056,#7057,#4248,.T.);
#8635=EDGE_CURVE('',#7010,#7057,#4249,.T.);
#8636=EDGE_CURVE('',#7030,#7058,#4250,.T.);
#8637=EDGE_CURVE('',#7058,#7059,#4251,.T.);
#8638=EDGE_CURVE('',#7059,#7051,#4252,.T.);
#8639=EDGE_CURVE('',#7003,#7060,#4253,.T.);
#8640=EDGE_CURVE('',#7060,#7061,#4254,.T.);
#8641=EDGE_CURVE('',#7061,#7062,#4255,.T.);
#8642=EDGE_CURVE('',#7062,#7036,#4256,.T.);
#8643=EDGE_CURVE('',#7063,#7063,#6239,.T.);
#8644=EDGE_CURVE('',#7063,#7050,#4257,.T.);
#8645=EDGE_CURVE('',#7064,#7064,#6240,.T.);
#8646=EDGE_CURVE('',#7064,#7049,#4258,.T.);
#8647=EDGE_CURVE('',#7034,#7065,#4259,.T.);
#8648=EDGE_CURVE('',#7065,#7065,#6241,.T.);
#8649=EDGE_CURVE('',#7033,#7066,#4260,.T.);
#8650=EDGE_CURVE('',#7066,#7066,#6242,.T.);
#8651=EDGE_CURVE('',#7067,#7068,#4261,.T.);
#8652=EDGE_CURVE('',#7067,#7062,#6243,.T.);
#8653=EDGE_CURVE('',#7068,#7061,#6244,.T.);
#8654=EDGE_CURVE('',#7037,#7067,#4262,.T.);
#8655=EDGE_CURVE('',#7069,#7060,#6245,.T.);
#8656=EDGE_CURVE('',#7068,#7069,#4263,.T.);
#8657=EDGE_CURVE('',#7070,#7029,#4264,.T.);
#8658=EDGE_CURVE('',#7070,#7058,#6246,.T.);
#8659=EDGE_CURVE('',#7071,#7070,#4265,.T.);
#8660=EDGE_CURVE('',#7059,#7071,#6247,.T.);
#8661=EDGE_CURVE('',#7052,#7071,#4266,.T.);
#8662=EDGE_CURVE('',#7028,#7072,#4267,.T.);
#8663=EDGE_CURVE('',#7072,#7073,#4268,.T.);
#8664=EDGE_CURVE('',#7073,#7053,#4269,.T.);
#8665=EDGE_CURVE('',#7069,#7074,#4270,.T.);
#8666=EDGE_CURVE('',#7074,#7075,#4271,.T.);
#8667=EDGE_CURVE('',#7075,#7076,#4272,.T.);
#8668=EDGE_CURVE('',#7076,#7038,#4273,.T.);
#8669=EDGE_CURVE('',#7077,#7077,#6248,.T.);
#8670=EDGE_CURVE('',#7077,#7047,#4274,.T.);
#8671=EDGE_CURVE('',#7078,#7078,#6249,.T.);
#8672=EDGE_CURVE('',#7078,#7048,#4275,.T.);
#8673=EDGE_CURVE('',#7031,#7079,#4276,.T.);
#8674=EDGE_CURVE('',#7079,#7079,#6250,.T.);
#8675=EDGE_CURVE('',#7032,#7080,#4277,.T.);
#8676=EDGE_CURVE('',#7080,#7080,#6251,.T.);
#8677=EDGE_CURVE('',#7081,#7076,#6252,.T.);
#8678=EDGE_CURVE('',#7039,#7081,#4278,.T.);
#8679=EDGE_CURVE('',#7082,#7075,#6253,.T.);
#8680=EDGE_CURVE('',#7081,#7082,#4279,.T.);
#8681=EDGE_CURVE('',#7083,#7027,#4280,.T.);
#8682=EDGE_CURVE('',#7083,#7072,#6254,.T.);
#8683=EDGE_CURVE('',#7084,#7083,#4281,.T.);
#8684=EDGE_CURVE('',#7073,#7084,#6255,.T.);
#8685=EDGE_CURVE('',#7054,#7084,#4282,.T.);
#8686=EDGE_CURVE('',#7085,#7074,#6256,.T.);
#8687=EDGE_CURVE('',#7082,#7085,#4283,.T.);
#8688=EDGE_CURVE('',#7011,#7086,#4284,.T.);
#8689=EDGE_CURVE('',#7086,#7087,#4285,.T.);
#8690=EDGE_CURVE('',#7088,#7087,#4286,.T.);
#8691=EDGE_CURVE('',#7085,#7088,#4287,.T.);
#8692=EDGE_CURVE('',#7088,#7055,#4288,.T.);
#8693=EDGE_CURVE('',#7040,#7026,#4289,.T.);
#8694=EDGE_CURVE('',#7089,#7089,#6257,.T.);
#8695=EDGE_CURVE('',#7090,#7090,#6258,.T.);
#8696=EDGE_CURVE('',#7091,#7091,#6259,.T.);
#8697=EDGE_CURVE('',#7092,#7092,#6260,.T.);
#8698=EDGE_CURVE('',#7093,#7093,#6261,.T.);
#8699=EDGE_CURVE('',#7012,#7094,#4290,.T.);
#8700=EDGE_CURVE('',#7094,#7094,#6262,.T.);
#8701=EDGE_CURVE('',#7016,#7095,#4291,.T.);
#8702=EDGE_CURVE('',#7095,#7095,#6263,.T.);
#8703=EDGE_CURVE('',#7089,#7096,#4292,.T.);
#8704=EDGE_CURVE('',#7096,#7096,#6264,.T.);
#8705=EDGE_CURVE('',#7093,#7097,#4293,.T.);
#8706=EDGE_CURVE('',#7097,#7097,#6265,.T.);
#8707=EDGE_CURVE('',#7013,#7098,#4294,.T.);
#8708=EDGE_CURVE('',#7098,#7098,#6266,.T.);
#8709=EDGE_CURVE('',#7090,#7099,#4295,.T.);
#8710=EDGE_CURVE('',#7099,#7099,#6267,.T.);
#8711=EDGE_CURVE('',#7091,#7100,#4296,.T.);
#8712=EDGE_CURVE('',#7100,#7100,#6268,.T.);
#8713=EDGE_CURVE('',#7092,#7101,#4297,.T.);
#8714=EDGE_CURVE('',#7101,#7101,#6269,.T.);
#8715=EDGE_CURVE('',#7014,#7102,#4298,.T.);
#8716=EDGE_CURVE('',#7102,#7102,#6270,.T.);
#8717=EDGE_CURVE('',#7015,#7103,#4299,.T.);
#8718=EDGE_CURVE('',#7103,#7103,#6271,.T.);
#8719=EDGE_CURVE('',#7020,#7046,#4300,.T.);
#8720=EDGE_CURVE('',#7021,#7045,#4301,.T.);
#8721=EDGE_CURVE('',#7041,#7025,#4302,.T.);
#8722=EDGE_CURVE('',#7042,#7024,#4303,.T.);
#8723=EDGE_CURVE('',#7043,#7023,#4304,.T.);
#8724=EDGE_CURVE('',#7057,#7086,#4305,.T.);
#8725=EDGE_CURVE('',#7087,#7056,#4306,.T.);
#8726=EDGE_CURVE('',#7022,#7044,#4307,.T.);
#10951=ORIENTED_EDGE('',*,*,#8529,.F.);
#10952=ORIENTED_EDGE('',*,*,#8530,.T.);
#10953=ORIENTED_EDGE('',*,*,#8531,.F.);
#10954=ORIENTED_EDGE('',*,*,#8530,.F.);
#10955=ORIENTED_EDGE('',*,*,#8532,.F.);
#10956=ORIENTED_EDGE('',*,*,#8533,.T.);
#10957=ORIENTED_EDGE('',*,*,#8534,.F.);
#10958=ORIENTED_EDGE('',*,*,#8533,.F.);
#10959=ORIENTED_EDGE('',*,*,#8535,.F.);
#10960=ORIENTED_EDGE('',*,*,#8536,.T.);
#10961=ORIENTED_EDGE('',*,*,#8537,.F.);
#10962=ORIENTED_EDGE('',*,*,#8536,.F.);
#10963=ORIENTED_EDGE('',*,*,#8538,.F.);
#10964=ORIENTED_EDGE('',*,*,#8539,.T.);
#10965=ORIENTED_EDGE('',*,*,#8540,.F.);
#10966=ORIENTED_EDGE('',*,*,#8539,.F.);
#10967=ORIENTED_EDGE('',*,*,#8541,.F.);
#10968=ORIENTED_EDGE('',*,*,#8542,.T.);
#10969=ORIENTED_EDGE('',*,*,#8543,.F.);
#10970=ORIENTED_EDGE('',*,*,#8544,.F.);
#10971=ORIENTED_EDGE('',*,*,#8545,.F.);
#10972=ORIENTED_EDGE('',*,*,#8544,.T.);
#10973=ORIENTED_EDGE('',*,*,#8546,.F.);
#10974=ORIENTED_EDGE('',*,*,#8547,.F.);
#10975=ORIENTED_EDGE('',*,*,#8548,.F.);
#10976=ORIENTED_EDGE('',*,*,#8547,.T.);
#10977=ORIENTED_EDGE('',*,*,#8549,.F.);
#10978=ORIENTED_EDGE('',*,*,#8550,.F.);
#10979=ORIENTED_EDGE('',*,*,#8551,.F.);
#10980=ORIENTED_EDGE('',*,*,#8550,.T.);
#10981=ORIENTED_EDGE('',*,*,#8552,.F.);
#10982=ORIENTED_EDGE('',*,*,#8542,.F.);
#10983=ORIENTED_EDGE('',*,*,#8553,.F.);
#10984=ORIENTED_EDGE('',*,*,#8554,.T.);
#10985=ORIENTED_EDGE('',*,*,#8555,.F.);
#10986=ORIENTED_EDGE('',*,*,#8554,.F.);
#10987=ORIENTED_EDGE('',*,*,#8553,.T.);
#10988=ORIENTED_EDGE('',*,*,#8556,.F.);
#10989=ORIENTED_EDGE('',*,*,#8557,.T.);
#10990=ORIENTED_EDGE('',*,*,#8558,.F.);
#10991=ORIENTED_EDGE('',*,*,#8557,.F.);
#10992=ORIENTED_EDGE('',*,*,#8556,.T.);
#10993=ORIENTED_EDGE('',*,*,#8559,.F.);
#10994=ORIENTED_EDGE('',*,*,#8560,.T.);
#10995=ORIENTED_EDGE('',*,*,#8561,.T.);
#10996=ORIENTED_EDGE('',*,*,#8560,.F.);
#10997=ORIENTED_EDGE('',*,*,#8561,.F.);
#10998=ORIENTED_EDGE('',*,*,#8562,.F.);
#10999=ORIENTED_EDGE('',*,*,#8563,.T.);
#11000=ORIENTED_EDGE('',*,*,#8564,.T.);
#11001=ORIENTED_EDGE('',*,*,#8563,.F.);
#11002=ORIENTED_EDGE('',*,*,#8564,.F.);
#11003=ORIENTED_EDGE('',*,*,#8565,.F.);
#11004=ORIENTED_EDGE('',*,*,#8566,.T.);
#11005=ORIENTED_EDGE('',*,*,#8567,.F.);
#11006=ORIENTED_EDGE('',*,*,#8568,.F.);
#11007=ORIENTED_EDGE('',*,*,#8569,.F.);
#11008=ORIENTED_EDGE('',*,*,#8570,.F.);
#11009=ORIENTED_EDGE('',*,*,#8571,.F.);
#11010=ORIENTED_EDGE('',*,*,#8566,.F.);
#11011=ORIENTED_EDGE('',*,*,#8568,.T.);
#11012=ORIENTED_EDGE('',*,*,#8572,.F.);
#11013=ORIENTED_EDGE('',*,*,#8573,.F.);
#11014=ORIENTED_EDGE('',*,*,#8574,.F.);
#11015=ORIENTED_EDGE('',*,*,#8567,.T.);
#11016=ORIENTED_EDGE('',*,*,#8571,.T.);
#11017=ORIENTED_EDGE('',*,*,#8575,.F.);
#11018=ORIENTED_EDGE('',*,*,#8576,.F.);
#11019=ORIENTED_EDGE('',*,*,#8577,.F.);
#11020=ORIENTED_EDGE('',*,*,#8578,.T.);
#11021=ORIENTED_EDGE('',*,*,#8579,.T.);
#11022=ORIENTED_EDGE('',*,*,#8580,.T.);
#11023=ORIENTED_EDGE('',*,*,#8581,.T.);
#11024=ORIENTED_EDGE('',*,*,#8582,.T.);
#11025=ORIENTED_EDGE('',*,*,#8583,.T.);
#11026=ORIENTED_EDGE('',*,*,#8572,.T.);
#11027=ORIENTED_EDGE('',*,*,#8584,.T.);
#11028=ORIENTED_EDGE('',*,*,#8585,.T.);
#11029=ORIENTED_EDGE('',*,*,#8586,.T.);
#11030=ORIENTED_EDGE('',*,*,#8587,.T.);
#11031=ORIENTED_EDGE('',*,*,#8588,.T.);
#11032=ORIENTED_EDGE('',*,*,#8589,.F.);
#11033=ORIENTED_EDGE('',*,*,#8590,.T.);
#11034=ORIENTED_EDGE('',*,*,#8578,.F.);
#11035=ORIENTED_EDGE('',*,*,#8591,.F.);
#11036=ORIENTED_EDGE('',*,*,#8592,.F.);
#11037=ORIENTED_EDGE('',*,*,#8593,.F.);
#11038=ORIENTED_EDGE('',*,*,#8579,.F.);
#11039=ORIENTED_EDGE('',*,*,#8590,.F.);
#11040=ORIENTED_EDGE('',*,*,#8591,.T.);
#11041=ORIENTED_EDGE('',*,*,#8577,.T.);
#11042=ORIENTED_EDGE('',*,*,#8594,.T.);
#11043=ORIENTED_EDGE('',*,*,#8595,.F.);
#11044=ORIENTED_EDGE('',*,*,#8596,.T.);
#11045=ORIENTED_EDGE('',*,*,#8597,.F.);
#11046=ORIENTED_EDGE('',*,*,#8598,.F.);
#11047=ORIENTED_EDGE('',*,*,#8599,.F.);
#11048=ORIENTED_EDGE('',*,*,#8600,.F.);
#11049=ORIENTED_EDGE('',*,*,#8601,.T.);
#11050=ORIENTED_EDGE('',*,*,#8602,.T.);
#11051=ORIENTED_EDGE('',*,*,#8603,.T.);
#11052=ORIENTED_EDGE('',*,*,#8604,.T.);
#11053=ORIENTED_EDGE('',*,*,#8605,.T.);
#11054=ORIENTED_EDGE('',*,*,#8559,.T.);
#11055=ORIENTED_EDGE('',*,*,#8562,.T.);
#11056=ORIENTED_EDGE('',*,*,#8606,.T.);
#11057=ORIENTED_EDGE('',*,*,#8607,.T.);
#11058=ORIENTED_EDGE('',*,*,#8608,.T.);
#11059=ORIENTED_EDGE('',*,*,#8609,.T.);
#11060=ORIENTED_EDGE('',*,*,#8593,.T.);
#11061=ORIENTED_EDGE('',*,*,#8610,.F.);
#11062=ORIENTED_EDGE('',*,*,#8611,.F.);
#11063=ORIENTED_EDGE('',*,*,#8580,.F.);
#11064=ORIENTED_EDGE('',*,*,#8570,.T.);
#11065=ORIENTED_EDGE('',*,*,#8612,.T.);
#11066=ORIENTED_EDGE('',*,*,#8613,.T.);
#11067=ORIENTED_EDGE('',*,*,#8614,.T.);
#11068=ORIENTED_EDGE('',*,*,#8615,.T.);
#11069=ORIENTED_EDGE('',*,*,#8616,.T.);
#11070=ORIENTED_EDGE('',*,*,#8617,.T.);
#11071=ORIENTED_EDGE('',*,*,#8618,.F.);
#11072=ORIENTED_EDGE('',*,*,#8619,.T.);
#11073=ORIENTED_EDGE('',*,*,#8620,.F.);
#11074=ORIENTED_EDGE('',*,*,#8621,.F.);
#11075=ORIENTED_EDGE('',*,*,#8622,.F.);
#11076=ORIENTED_EDGE('',*,*,#8623,.F.);
#11077=ORIENTED_EDGE('',*,*,#8575,.T.);
#11078=ORIENTED_EDGE('',*,*,#8555,.T.);
#11079=ORIENTED_EDGE('',*,*,#8558,.T.);
#11080=ORIENTED_EDGE('',*,*,#8624,.T.);
#11081=ORIENTED_EDGE('',*,*,#8625,.T.);
#11082=ORIENTED_EDGE('',*,*,#8626,.T.);
#11083=ORIENTED_EDGE('',*,*,#8627,.T.);
#11084=ORIENTED_EDGE('',*,*,#8611,.T.);
#11085=ORIENTED_EDGE('',*,*,#8628,.F.);
#11086=ORIENTED_EDGE('',*,*,#8629,.T.);
#11087=ORIENTED_EDGE('',*,*,#8630,.F.);
#11088=ORIENTED_EDGE('',*,*,#8631,.T.);
#11089=ORIENTED_EDGE('',*,*,#8632,.F.);
#11090=ORIENTED_EDGE('',*,*,#8633,.T.);
#11091=ORIENTED_EDGE('',*,*,#8634,.T.);
#11092=ORIENTED_EDGE('',*,*,#8635,.F.);
#11093=ORIENTED_EDGE('',*,*,#8581,.F.);
#11094=ORIENTED_EDGE('',*,*,#8589,.T.);
#11095=ORIENTED_EDGE('',*,*,#8605,.F.);
#11096=ORIENTED_EDGE('',*,*,#8636,.T.);
#11097=ORIENTED_EDGE('',*,*,#8637,.T.);
#11098=ORIENTED_EDGE('',*,*,#8638,.T.);
#11099=ORIENTED_EDGE('',*,*,#8628,.T.);
#11100=ORIENTED_EDGE('',*,*,#8610,.T.);
#11101=ORIENTED_EDGE('',*,*,#8592,.T.);
#11102=ORIENTED_EDGE('',*,*,#8565,.T.);
#11103=ORIENTED_EDGE('',*,*,#8574,.T.);
#11104=ORIENTED_EDGE('',*,*,#8639,.T.);
#11105=ORIENTED_EDGE('',*,*,#8640,.T.);
#11106=ORIENTED_EDGE('',*,*,#8641,.T.);
#11107=ORIENTED_EDGE('',*,*,#8642,.T.);
#11108=ORIENTED_EDGE('',*,*,#8612,.F.);
#11109=ORIENTED_EDGE('',*,*,#8569,.T.);
#11110=ORIENTED_EDGE('',*,*,#8643,.F.);
#11111=ORIENTED_EDGE('',*,*,#8644,.T.);
#11112=ORIENTED_EDGE('',*,*,#8627,.F.);
#11113=ORIENTED_EDGE('',*,*,#8644,.F.);
#11114=ORIENTED_EDGE('',*,*,#8643,.T.);
#11115=ORIENTED_EDGE('',*,*,#8645,.F.);
#11116=ORIENTED_EDGE('',*,*,#8646,.T.);
#11117=ORIENTED_EDGE('',*,*,#8626,.F.);
#11118=ORIENTED_EDGE('',*,*,#8646,.F.);
#11119=ORIENTED_EDGE('',*,*,#8645,.T.);
#11120=ORIENTED_EDGE('',*,*,#8609,.F.);
#11121=ORIENTED_EDGE('',*,*,#8647,.T.);
#11122=ORIENTED_EDGE('',*,*,#8648,.T.);
#11123=ORIENTED_EDGE('',*,*,#8647,.F.);
#11124=ORIENTED_EDGE('',*,*,#8648,.F.);
#11125=ORIENTED_EDGE('',*,*,#8608,.F.);
#11126=ORIENTED_EDGE('',*,*,#8649,.T.);
#11127=ORIENTED_EDGE('',*,*,#8650,.T.);
#11128=ORIENTED_EDGE('',*,*,#8649,.F.);
#11129=ORIENTED_EDGE('',*,*,#8650,.F.);
#11130=ORIENTED_EDGE('',*,*,#8651,.F.);
#11131=ORIENTED_EDGE('',*,*,#8652,.T.);
#11132=ORIENTED_EDGE('',*,*,#8641,.F.);
#11133=ORIENTED_EDGE('',*,*,#8653,.F.);
#11134=ORIENTED_EDGE('',*,*,#8654,.F.);
#11135=ORIENTED_EDGE('',*,*,#8613,.F.);
#11136=ORIENTED_EDGE('',*,*,#8642,.F.);
#11137=ORIENTED_EDGE('',*,*,#8652,.F.);
#11138=ORIENTED_EDGE('',*,*,#8653,.T.);
#11139=ORIENTED_EDGE('',*,*,#8640,.F.);
#11140=ORIENTED_EDGE('',*,*,#8655,.F.);
#11141=ORIENTED_EDGE('',*,*,#8656,.F.);
#11142=ORIENTED_EDGE('',*,*,#8657,.F.);
#11143=ORIENTED_EDGE('',*,*,#8658,.T.);
#11144=ORIENTED_EDGE('',*,*,#8636,.F.);
#11145=ORIENTED_EDGE('',*,*,#8604,.F.);
#11146=ORIENTED_EDGE('',*,*,#8659,.F.);
#11147=ORIENTED_EDGE('',*,*,#8660,.F.);
#11148=ORIENTED_EDGE('',*,*,#8637,.F.);
#11149=ORIENTED_EDGE('',*,*,#8658,.F.);
#11150=ORIENTED_EDGE('',*,*,#8660,.T.);
#11151=ORIENTED_EDGE('',*,*,#8661,.F.);
#11152=ORIENTED_EDGE('',*,*,#8629,.F.);
#11153=ORIENTED_EDGE('',*,*,#8638,.F.);
#11154=ORIENTED_EDGE('',*,*,#8657,.T.);
#11155=ORIENTED_EDGE('',*,*,#8603,.F.);
#11156=ORIENTED_EDGE('',*,*,#8662,.T.);
#11157=ORIENTED_EDGE('',*,*,#8663,.T.);
#11158=ORIENTED_EDGE('',*,*,#8664,.T.);
#11159=ORIENTED_EDGE('',*,*,#8630,.T.);
#11160=ORIENTED_EDGE('',*,*,#8661,.T.);
#11161=ORIENTED_EDGE('',*,*,#8659,.T.);
#11162=ORIENTED_EDGE('',*,*,#8651,.T.);
#11163=ORIENTED_EDGE('',*,*,#8656,.T.);
#11164=ORIENTED_EDGE('',*,*,#8665,.T.);
#11165=ORIENTED_EDGE('',*,*,#8666,.T.);
#11166=ORIENTED_EDGE('',*,*,#8667,.T.);
#11167=ORIENTED_EDGE('',*,*,#8668,.T.);
#11168=ORIENTED_EDGE('',*,*,#8614,.F.);
#11169=ORIENTED_EDGE('',*,*,#8654,.T.);
#11170=ORIENTED_EDGE('',*,*,#8669,.F.);
#11171=ORIENTED_EDGE('',*,*,#8670,.T.);
#11172=ORIENTED_EDGE('',*,*,#8624,.F.);
#11173=ORIENTED_EDGE('',*,*,#8670,.F.);
#11174=ORIENTED_EDGE('',*,*,#8669,.T.);
#11175=ORIENTED_EDGE('',*,*,#8671,.F.);
#11176=ORIENTED_EDGE('',*,*,#8672,.T.);
#11177=ORIENTED_EDGE('',*,*,#8625,.F.);
#11178=ORIENTED_EDGE('',*,*,#8672,.F.);
#11179=ORIENTED_EDGE('',*,*,#8671,.T.);
#11180=ORIENTED_EDGE('',*,*,#8606,.F.);
#11181=ORIENTED_EDGE('',*,*,#8673,.T.);
#11182=ORIENTED_EDGE('',*,*,#8674,.T.);
#11183=ORIENTED_EDGE('',*,*,#8673,.F.);
#11184=ORIENTED_EDGE('',*,*,#8674,.F.);
#11185=ORIENTED_EDGE('',*,*,#8607,.F.);
#11186=ORIENTED_EDGE('',*,*,#8675,.T.);
#11187=ORIENTED_EDGE('',*,*,#8676,.T.);
#11188=ORIENTED_EDGE('',*,*,#8675,.F.);
#11189=ORIENTED_EDGE('',*,*,#8676,.F.);
#11190=ORIENTED_EDGE('',*,*,#8668,.F.);
#11191=ORIENTED_EDGE('',*,*,#8677,.F.);
#11192=ORIENTED_EDGE('',*,*,#8678,.F.);
#11193=ORIENTED_EDGE('',*,*,#8615,.F.);
#11194=ORIENTED_EDGE('',*,*,#8667,.F.);
#11195=ORIENTED_EDGE('',*,*,#8679,.F.);
#11196=ORIENTED_EDGE('',*,*,#8680,.F.);
#11197=ORIENTED_EDGE('',*,*,#8677,.T.);
#11198=ORIENTED_EDGE('',*,*,#8681,.F.);
#11199=ORIENTED_EDGE('',*,*,#8682,.T.);
#11200=ORIENTED_EDGE('',*,*,#8662,.F.);
#11201=ORIENTED_EDGE('',*,*,#8602,.F.);
#11202=ORIENTED_EDGE('',*,*,#8683,.F.);
#11203=ORIENTED_EDGE('',*,*,#8684,.F.);
#11204=ORIENTED_EDGE('',*,*,#8663,.F.);
#11205=ORIENTED_EDGE('',*,*,#8682,.F.);
#11206=ORIENTED_EDGE('',*,*,#8684,.T.);
#11207=ORIENTED_EDGE('',*,*,#8685,.F.);
#11208=ORIENTED_EDGE('',*,*,#8631,.F.);
#11209=ORIENTED_EDGE('',*,*,#8664,.F.);
#11210=ORIENTED_EDGE('',*,*,#8679,.T.);
#11211=ORIENTED_EDGE('',*,*,#8666,.F.);
#11212=ORIENTED_EDGE('',*,*,#8686,.F.);
#11213=ORIENTED_EDGE('',*,*,#8687,.F.);
#11214=ORIENTED_EDGE('',*,*,#8573,.T.);
#11215=ORIENTED_EDGE('',*,*,#8583,.F.);
#11216=ORIENTED_EDGE('',*,*,#8688,.T.);
#11217=ORIENTED_EDGE('',*,*,#8689,.T.);
#11218=ORIENTED_EDGE('',*,*,#8690,.F.);
#11219=ORIENTED_EDGE('',*,*,#8691,.F.);
#11220=ORIENTED_EDGE('',*,*,#8686,.T.);
#11221=ORIENTED_EDGE('',*,*,#8665,.F.);
#11222=ORIENTED_EDGE('',*,*,#8655,.T.);
#11223=ORIENTED_EDGE('',*,*,#8639,.F.);
#11224=ORIENTED_EDGE('',*,*,#8680,.T.);
#11225=ORIENTED_EDGE('',*,*,#8687,.T.);
#11226=ORIENTED_EDGE('',*,*,#8691,.T.);
#11227=ORIENTED_EDGE('',*,*,#8692,.T.);
#11228=ORIENTED_EDGE('',*,*,#8632,.T.);
#11229=ORIENTED_EDGE('',*,*,#8685,.T.);
#11230=ORIENTED_EDGE('',*,*,#8683,.T.);
#11231=ORIENTED_EDGE('',*,*,#8681,.T.);
#11232=ORIENTED_EDGE('',*,*,#8601,.F.);
#11233=ORIENTED_EDGE('',*,*,#8693,.F.);
#11234=ORIENTED_EDGE('',*,*,#8616,.F.);
#11235=ORIENTED_EDGE('',*,*,#8678,.T.);
#11236=ORIENTED_EDGE('',*,*,#8694,.T.);
#11237=ORIENTED_EDGE('',*,*,#8695,.T.);
#11238=ORIENTED_EDGE('',*,*,#8696,.T.);
#11239=ORIENTED_EDGE('',*,*,#8697,.T.);
#11240=ORIENTED_EDGE('',*,*,#8698,.T.);
#11241=ORIENTED_EDGE('',*,*,#8584,.F.);
#11242=ORIENTED_EDGE('',*,*,#8699,.T.);
#11243=ORIENTED_EDGE('',*,*,#8700,.T.);
#11244=ORIENTED_EDGE('',*,*,#8699,.F.);
#11245=ORIENTED_EDGE('',*,*,#8700,.F.);
#11246=ORIENTED_EDGE('',*,*,#8588,.F.);
#11247=ORIENTED_EDGE('',*,*,#8701,.T.);
#11248=ORIENTED_EDGE('',*,*,#8702,.T.);
#11249=ORIENTED_EDGE('',*,*,#8701,.F.);
#11250=ORIENTED_EDGE('',*,*,#8702,.F.);
#11251=ORIENTED_EDGE('',*,*,#8694,.F.);
#11252=ORIENTED_EDGE('',*,*,#8703,.T.);
#11253=ORIENTED_EDGE('',*,*,#8704,.T.);
#11254=ORIENTED_EDGE('',*,*,#8703,.F.);
#11255=ORIENTED_EDGE('',*,*,#8704,.F.);
#11256=ORIENTED_EDGE('',*,*,#8698,.F.);
#11257=ORIENTED_EDGE('',*,*,#8705,.T.);
#11258=ORIENTED_EDGE('',*,*,#8706,.T.);
#11259=ORIENTED_EDGE('',*,*,#8705,.F.);
#11260=ORIENTED_EDGE('',*,*,#8706,.F.);
#11261=ORIENTED_EDGE('',*,*,#8585,.F.);
#11262=ORIENTED_EDGE('',*,*,#8707,.T.);
#11263=ORIENTED_EDGE('',*,*,#8708,.F.);
#11264=ORIENTED_EDGE('',*,*,#8707,.F.);
#11265=ORIENTED_EDGE('',*,*,#8695,.F.);
#11266=ORIENTED_EDGE('',*,*,#8709,.T.);
#11267=ORIENTED_EDGE('',*,*,#8710,.F.);
#11268=ORIENTED_EDGE('',*,*,#8709,.F.);
#11269=ORIENTED_EDGE('',*,*,#8696,.F.);
#11270=ORIENTED_EDGE('',*,*,#8711,.T.);
#11271=ORIENTED_EDGE('',*,*,#8712,.F.);
#11272=ORIENTED_EDGE('',*,*,#8711,.F.);
#11273=ORIENTED_EDGE('',*,*,#8697,.F.);
#11274=ORIENTED_EDGE('',*,*,#8713,.T.);
#11275=ORIENTED_EDGE('',*,*,#8714,.F.);
#11276=ORIENTED_EDGE('',*,*,#8713,.F.);
#11277=ORIENTED_EDGE('',*,*,#8586,.F.);
#11278=ORIENTED_EDGE('',*,*,#8715,.T.);
#11279=ORIENTED_EDGE('',*,*,#8716,.F.);
#11280=ORIENTED_EDGE('',*,*,#8715,.F.);
#11281=ORIENTED_EDGE('',*,*,#8587,.F.);
#11282=ORIENTED_EDGE('',*,*,#8717,.T.);
#11283=ORIENTED_EDGE('',*,*,#8718,.F.);
#11284=ORIENTED_EDGE('',*,*,#8717,.F.);
#11285=ORIENTED_EDGE('',*,*,#8576,.T.);
#11286=ORIENTED_EDGE('',*,*,#8623,.T.);
#11287=ORIENTED_EDGE('',*,*,#8719,.F.);
#11288=ORIENTED_EDGE('',*,*,#8594,.F.);
#11289=ORIENTED_EDGE('',*,*,#8720,.F.);
#11290=ORIENTED_EDGE('',*,*,#8595,.T.);
#11291=ORIENTED_EDGE('',*,*,#8719,.T.);
#11292=ORIENTED_EDGE('',*,*,#8622,.T.);
#11293=ORIENTED_EDGE('',*,*,#8708,.T.);
#11294=ORIENTED_EDGE('',*,*,#8716,.T.);
#11295=ORIENTED_EDGE('',*,*,#8718,.T.);
#11296=ORIENTED_EDGE('',*,*,#8693,.T.);
#11297=ORIENTED_EDGE('',*,*,#8600,.T.);
#11298=ORIENTED_EDGE('',*,*,#8721,.F.);
#11299=ORIENTED_EDGE('',*,*,#8617,.F.);
#11300=ORIENTED_EDGE('',*,*,#8721,.T.);
#11301=ORIENTED_EDGE('',*,*,#8599,.T.);
#11302=ORIENTED_EDGE('',*,*,#8722,.F.);
#11303=ORIENTED_EDGE('',*,*,#8618,.T.);
#11304=ORIENTED_EDGE('',*,*,#8710,.T.);
#11305=ORIENTED_EDGE('',*,*,#8712,.T.);
#11306=ORIENTED_EDGE('',*,*,#8714,.T.);
#11307=ORIENTED_EDGE('',*,*,#8722,.T.);
#11308=ORIENTED_EDGE('',*,*,#8598,.T.);
#11309=ORIENTED_EDGE('',*,*,#8723,.F.);
#11310=ORIENTED_EDGE('',*,*,#8619,.F.);
#11311=ORIENTED_EDGE('',*,*,#8582,.F.);
#11312=ORIENTED_EDGE('',*,*,#8635,.T.);
#11313=ORIENTED_EDGE('',*,*,#8724,.T.);
#11314=ORIENTED_EDGE('',*,*,#8688,.F.);
#11315=ORIENTED_EDGE('',*,*,#8692,.F.);
#11316=ORIENTED_EDGE('',*,*,#8690,.T.);
#11317=ORIENTED_EDGE('',*,*,#8725,.T.);
#11318=ORIENTED_EDGE('',*,*,#8633,.F.);
#11319=ORIENTED_EDGE('',*,*,#8725,.F.);
#11320=ORIENTED_EDGE('',*,*,#8689,.F.);
#11321=ORIENTED_EDGE('',*,*,#8724,.F.);
#11322=ORIENTED_EDGE('',*,*,#8634,.F.);
#11323=ORIENTED_EDGE('',*,*,#8548,.T.);
#11324=ORIENTED_EDGE('',*,*,#8551,.T.);
#11325=ORIENTED_EDGE('',*,*,#8541,.T.);
#11326=ORIENTED_EDGE('',*,*,#8545,.T.);
#11327=ORIENTED_EDGE('',*,*,#8538,.T.);
#11328=ORIENTED_EDGE('',*,*,#8535,.T.);
#11329=ORIENTED_EDGE('',*,*,#8532,.T.);
#11330=ORIENTED_EDGE('',*,*,#8529,.T.);
#11331=ORIENTED_EDGE('',*,*,#8720,.T.);
#11332=ORIENTED_EDGE('',*,*,#8621,.T.);
#11333=ORIENTED_EDGE('',*,*,#8726,.F.);
#11334=ORIENTED_EDGE('',*,*,#8596,.F.);
#11335=ORIENTED_EDGE('',*,*,#8723,.T.);
#11336=ORIENTED_EDGE('',*,*,#8597,.T.);
#11337=ORIENTED_EDGE('',*,*,#8726,.T.);
#11338=ORIENTED_EDGE('',*,*,#8620,.T.);
#11339=ORIENTED_EDGE('',*,*,#8549,.T.);
#11340=ORIENTED_EDGE('',*,*,#8546,.T.);
#11341=ORIENTED_EDGE('',*,*,#8543,.T.);
#11342=ORIENTED_EDGE('',*,*,#8552,.T.);
#11343=ORIENTED_EDGE('',*,*,#8540,.T.);
#11344=ORIENTED_EDGE('',*,*,#8537,.T.);
#11345=ORIENTED_EDGE('',*,*,#8534,.T.);
#11346=ORIENTED_EDGE('',*,*,#8531,.T.);
#14953=CYLINDRICAL_SURFACE('',#17007,0.164999999999999);
#14954=CYLINDRICAL_SURFACE('',#17010,0.165);
#14955=CYLINDRICAL_SURFACE('',#17013,0.165);
#14956=CYLINDRICAL_SURFACE('',#17016,0.164999999999999);
#14957=CYLINDRICAL_SURFACE('',#17023,0.164999999999999);
#14958=CYLINDRICAL_SURFACE('',#17027,0.164999999999999);
#14959=CYLINDRICAL_SURFACE('',#17031,0.164999999999999);
#14960=CYLINDRICAL_SURFACE('',#17035,0.164999999999999);
#14961=CYLINDRICAL_SURFACE('',#17042,2.35);
#14962=CYLINDRICAL_SURFACE('',#17044,1.9);
#14963=CYLINDRICAL_SURFACE('',#17052,2.35);
#14964=CYLINDRICAL_SURFACE('',#17064,1.9);
#14965=CYLINDRICAL_SURFACE('',#17078,0.165);
#14966=CYLINDRICAL_SURFACE('',#17081,0.165);
#14967=CYLINDRICAL_SURFACE('',#17084,0.165);
#14968=CYLINDRICAL_SURFACE('',#17087,0.165);
#14969=CYLINDRICAL_SURFACE('',#17093,2.35);
#14970=CYLINDRICAL_SURFACE('',#17094,1.9);
#14971=CYLINDRICAL_SURFACE('',#17096,2.35);
#14972=CYLINDRICAL_SURFACE('',#17100,1.9);
#14973=CYLINDRICAL_SURFACE('',#17103,0.165);
#14974=CYLINDRICAL_SURFACE('',#17106,0.165);
#14975=CYLINDRICAL_SURFACE('',#17109,0.165);
#14976=CYLINDRICAL_SURFACE('',#17112,0.165);
#14977=CYLINDRICAL_SURFACE('',#17115,1.6);
#14978=CYLINDRICAL_SURFACE('',#17119,1.6);
#14979=CYLINDRICAL_SURFACE('',#17123,1.2);
#14980=CYLINDRICAL_SURFACE('',#17124,1.2);
#14981=CYLINDRICAL_SURFACE('',#17133,0.149999999999999);
#14982=CYLINDRICAL_SURFACE('',#17136,0.149999999999999);
#14983=CYLINDRICAL_SURFACE('',#17139,0.15);
#14984=CYLINDRICAL_SURFACE('',#17142,0.15);
#14985=CYLINDRICAL_SURFACE('',#17145,0.329999999999998);
#14986=CYLINDRICAL_SURFACE('',#17147,0.33);
#14987=CYLINDRICAL_SURFACE('',#17149,0.33);
#14988=CYLINDRICAL_SURFACE('',#17151,0.33);
#14989=CYLINDRICAL_SURFACE('',#17153,0.329999999999998);
#14990=CYLINDRICAL_SURFACE('',#17155,0.329999999999998);
#15307=ADVANCED_FACE('',(#2100),#14953,.F.);
#15308=ADVANCED_FACE('',(#2101),#14954,.F.);
#15309=ADVANCED_FACE('',(#2102),#14955,.F.);
#15310=ADVANCED_FACE('',(#2103),#14956,.F.);
#15311=ADVANCED_FACE('',(#2104),#1654,.F.);
#15312=ADVANCED_FACE('',(#2105),#1655,.F.);
#15313=ADVANCED_FACE('',(#2106),#1656,.F.);
#15314=ADVANCED_FACE('',(#2107),#1657,.F.);
#15315=ADVANCED_FACE('',(#2108),#14957,.F.);
#15316=ADVANCED_FACE('',(#2109),#1658,.T.);
#15317=ADVANCED_FACE('',(#2110),#14958,.F.);
#15318=ADVANCED_FACE('',(#2111),#1659,.T.);
#15319=ADVANCED_FACE('',(#2112),#14959,.F.);
#15320=ADVANCED_FACE('',(#2113),#1660,.F.);
#15321=ADVANCED_FACE('',(#2114),#14960,.F.);
#15322=ADVANCED_FACE('',(#2115),#1661,.F.);
#15323=ADVANCED_FACE('',(#2116),#1662,.T.);
#15324=ADVANCED_FACE('',(#2117),#14961,.F.);
#15325=ADVANCED_FACE('',(#2118),#14962,.F.);
#15326=ADVANCED_FACE('',(#2119,#1422,#1423,#1424,#1425,#1426),#1663,.F.);
#15327=ADVANCED_FACE('',(#2120),#14963,.F.);
#15328=ADVANCED_FACE('',(#2121),#1664,.F.);
#15329=ADVANCED_FACE('',(#2122,#1427,#1428,#1429,#1430,#1431,#1432),#1665,
 .T.);
#15330=ADVANCED_FACE('',(#2123),#14964,.F.);
#15331=ADVANCED_FACE('',(#2124,#1433,#1434,#1435,#1436,#1437,#1438),#1666,
 .T.);
#15332=ADVANCED_FACE('',(#2125),#1667,.F.);
#15333=ADVANCED_FACE('',(#2126),#1668,.F.);
#15334=ADVANCED_FACE('',(#2127),#1669,.F.);
#15335=ADVANCED_FACE('',(#2128),#14965,.F.);
#15336=ADVANCED_FACE('',(#2129),#1670,.T.);
#15337=ADVANCED_FACE('',(#2130),#14966,.F.);
#15338=ADVANCED_FACE('',(#2131),#1671,.T.);
#15339=ADVANCED_FACE('',(#2132),#14967,.F.);
#15340=ADVANCED_FACE('',(#2133),#1672,.F.);
#15341=ADVANCED_FACE('',(#2134),#14968,.F.);
#15342=ADVANCED_FACE('',(#2135),#1673,.F.);
#15343=ADVANCED_FACE('',(#2136),#1674,.T.);
#15344=ADVANCED_FACE('',(#2137),#14969,.F.);
#15345=ADVANCED_FACE('',(#2138),#14970,.F.);
#15346=ADVANCED_FACE('',(#2139),#14971,.F.);
#15347=ADVANCED_FACE('',(#2140),#1675,.F.);
#15348=ADVANCED_FACE('',(#2141),#14972,.F.);
#15349=ADVANCED_FACE('',(#2142),#1676,.F.);
#15350=ADVANCED_FACE('',(#2143),#1677,.F.);
#15351=ADVANCED_FACE('',(#2144),#14973,.F.);
#15352=ADVANCED_FACE('',(#2145),#1678,.T.);
#15353=ADVANCED_FACE('',(#2146),#14974,.F.);
#15354=ADVANCED_FACE('',(#2147),#1679,.T.);
#15355=ADVANCED_FACE('',(#2148),#14975,.F.);
#15356=ADVANCED_FACE('',(#2149),#1680,.F.);
#15357=ADVANCED_FACE('',(#2150),#14976,.F.);
#15358=ADVANCED_FACE('',(#2151),#1681,.F.);
#15359=ADVANCED_FACE('',(#2152),#14977,.F.);
#15360=ADVANCED_FACE('',(#2153),#1682,.T.);
#15361=ADVANCED_FACE('',(#2154),#14978,.F.);
#15362=ADVANCED_FACE('',(#2155),#1683,.F.);
#15363=ADVANCED_FACE('',(#2156),#14979,.F.);
#15364=ADVANCED_FACE('',(#2157),#14980,.F.);
#15365=ADVANCED_FACE('',(#2158),#1684,.F.);
#15366=ADVANCED_FACE('',(#2159,#1439,#1440,#1441,#1442,#1443),#1685,.F.);
#15367=ADVANCED_FACE('',(#2160),#14981,.F.);
#15368=ADVANCED_FACE('',(#2161),#1686,.F.);
#15369=ADVANCED_FACE('',(#2162),#14982,.F.);
#15370=ADVANCED_FACE('',(#2163),#1687,.F.);
#15371=ADVANCED_FACE('',(#2164),#14983,.F.);
#15372=ADVANCED_FACE('',(#2165),#1688,.F.);
#15373=ADVANCED_FACE('',(#2166),#14984,.F.);
#15374=ADVANCED_FACE('',(#2167),#1689,.F.);
#15375=ADVANCED_FACE('',(#2168),#14985,.F.);
#15376=ADVANCED_FACE('',(#2169),#14986,.F.);
#15377=ADVANCED_FACE('',(#2170),#14987,.F.);
#15378=ADVANCED_FACE('',(#2171),#14988,.F.);
#15379=ADVANCED_FACE('',(#2172),#14989,.F.);
#15380=ADVANCED_FACE('',(#2173),#14990,.F.);
#15381=ADVANCED_FACE('',(#2174),#1690,.T.);
#15382=ADVANCED_FACE('',(#2175,#1444,#1445,#1446),#1691,.T.);
#15383=ADVANCED_FACE('',(#2176),#1692,.T.);
#15384=ADVANCED_FACE('',(#2177,#1447,#1448,#1449),#1693,.T.);
#15385=ADVANCED_FACE('',(#2178),#1694,.T.);
#15386=ADVANCED_FACE('',(#2179),#1695,.F.);
#15387=ADVANCED_FACE('',(#2180),#1696,.F.);
#15388=ADVANCED_FACE('',(#2181,#1450,#1451,#1452,#1453,#1454),#1697,.F.);
#15389=ADVANCED_FACE('',(#2182),#1698,.T.);
#15390=ADVANCED_FACE('',(#2183,#1455,#1456,#1457,#1458,#1459),#1699,.T.);
#16124=CLOSED_SHELL('',(#15307,#15308,#15309,#15310,#15311,#15312,#15313,
#15314,#15315,#15316,#15317,#15318,#15319,#15320,#15321,#15322,#15323,#15324,
#15325,#15326,#15327,#15328,#15329,#15330,#15331,#15332,#15333,#15334,#15335,
#15336,#15337,#15338,#15339,#15340,#15341,#15342,#15343,#15344,#15345,#15346,
#15347,#15348,#15349,#15350,#15351,#15352,#15353,#15354,#15355,#15356,#15357,
#15358,#15359,#15360,#15361,#15362,#15363,#15364,#15365,#15366,#15367,#15368,
#15369,#15370,#15371,#15372,#15373,#15374,#15375,#15376,#15377,#15378,#15379,
#15380,#15381,#15382,#15383,#15384,#15385,#15386,#15387,#15388,#15389,#15390));
#17006=AXIS2_PLACEMENT_3D('',#23246,#18976,#18977);
#17007=AXIS2_PLACEMENT_3D('',#23247,#18978,#18979);
#17008=AXIS2_PLACEMENT_3D('',#23249,#18980,#18981);
#17009=AXIS2_PLACEMENT_3D('',#23252,#18983,#18984);
#17010=AXIS2_PLACEMENT_3D('',#23253,#18985,#18986);
#17011=AXIS2_PLACEMENT_3D('',#23255,#18987,#18988);
#17012=AXIS2_PLACEMENT_3D('',#23258,#18990,#18991);
#17013=AXIS2_PLACEMENT_3D('',#23259,#18992,#18993);
#17014=AXIS2_PLACEMENT_3D('',#23261,#18994,#18995);
#17015=AXIS2_PLACEMENT_3D('',#23264,#18997,#18998);
#17016=AXIS2_PLACEMENT_3D('',#23265,#18999,#19000);
#17017=AXIS2_PLACEMENT_3D('',#23267,#19001,#19002);
#17018=AXIS2_PLACEMENT_3D('',#23270,#19004,#19005);
#17019=AXIS2_PLACEMENT_3D('',#23271,#19006,#19007);
#17020=AXIS2_PLACEMENT_3D('',#23280,#19012,#19013);
#17021=AXIS2_PLACEMENT_3D('',#23286,#19017,#19018);
#17022=AXIS2_PLACEMENT_3D('',#23292,#19022,#19023);
#17023=AXIS2_PLACEMENT_3D('',#23295,#19026,#19027);
#17024=AXIS2_PLACEMENT_3D('',#23297,#19028,#19029);
#17025=AXIS2_PLACEMENT_3D('',#23300,#19031,#19032);
#17026=AXIS2_PLACEMENT_3D('',#23301,#19033,#19034);
#17027=AXIS2_PLACEMENT_3D('',#23302,#19035,#19036);
#17028=AXIS2_PLACEMENT_3D('',#23304,#19037,#19038);
#17029=AXIS2_PLACEMENT_3D('',#23307,#19040,#19041);
#17030=AXIS2_PLACEMENT_3D('',#23308,#19042,#19043);
#17031=AXIS2_PLACEMENT_3D('',#23309,#19044,#19045);
#17032=AXIS2_PLACEMENT_3D('',#23311,#19046,#19047);
#17033=AXIS2_PLACEMENT_3D('',#23314,#19049,#19050);
#17034=AXIS2_PLACEMENT_3D('',#23315,#19051,#19052);
#17035=AXIS2_PLACEMENT_3D('',#23316,#19053,#19054);
#17036=AXIS2_PLACEMENT_3D('',#23318,#19055,#19056);
#17037=AXIS2_PLACEMENT_3D('',#23321,#19058,#19059);
#17038=AXIS2_PLACEMENT_3D('',#23322,#19060,#19061);
#17039=AXIS2_PLACEMENT_3D('',#23323,#19062,#19063);
#17040=AXIS2_PLACEMENT_3D('',#23328,#19065,#19066);
#17041=AXIS2_PLACEMENT_3D('',#23331,#19068,#19069);
#17042=AXIS2_PLACEMENT_3D('',#23332,#19070,#19071);
#17043=AXIS2_PLACEMENT_3D('',#23336,#19073,#19074);
#17044=AXIS2_PLACEMENT_3D('',#23338,#19076,#19077);
#17045=AXIS2_PLACEMENT_3D('',#23342,#19079,#19080);
#17046=AXIS2_PLACEMENT_3D('',#23344,#19082,#19083);
#17047=AXIS2_PLACEMENT_3D('',#23363,#19093,#19094);
#17048=AXIS2_PLACEMENT_3D('',#23365,#19095,#19096);
#17049=AXIS2_PLACEMENT_3D('',#23367,#19097,#19098);
#17050=AXIS2_PLACEMENT_3D('',#23369,#19099,#19100);
#17051=AXIS2_PLACEMENT_3D('',#23371,#19101,#19102);
#17052=AXIS2_PLACEMENT_3D('',#23372,#19103,#19104);
#17053=AXIS2_PLACEMENT_3D('',#23376,#19106,#19107);
#17054=AXIS2_PLACEMENT_3D('',#23377,#19108,#19109);
#17055=AXIS2_PLACEMENT_3D('',#23378,#19110,#19111);
#17056=AXIS2_PLACEMENT_3D('',#23381,#19113,#19114);
#17057=AXIS2_PLACEMENT_3D('',#23382,#19115,#19116);
#17058=AXIS2_PLACEMENT_3D('',#23400,#19125,#19126);
#17059=AXIS2_PLACEMENT_3D('',#23404,#19128,#19129);
#17060=AXIS2_PLACEMENT_3D('',#23407,#19131,#19132);
#17061=AXIS2_PLACEMENT_3D('',#23409,#19133,#19134);
#17062=AXIS2_PLACEMENT_3D('',#23411,#19135,#19136);
#17063=AXIS2_PLACEMENT_3D('',#23413,#19137,#19138);
#17064=AXIS2_PLACEMENT_3D('',#23414,#19139,#19140);
#17065=AXIS2_PLACEMENT_3D('',#23417,#19142,#19143);
#17066=AXIS2_PLACEMENT_3D('',#23418,#19144,#19145);
#17067=AXIS2_PLACEMENT_3D('',#23422,#19147,#19148);
#17068=AXIS2_PLACEMENT_3D('',#23426,#19150,#19151);
#17069=AXIS2_PLACEMENT_3D('',#23443,#19160,#19161);
#17070=AXIS2_PLACEMENT_3D('',#23445,#19162,#19163);
#17071=AXIS2_PLACEMENT_3D('',#23447,#19164,#19165);
#17072=AXIS2_PLACEMENT_3D('',#23449,#19166,#19167);
#17073=AXIS2_PLACEMENT_3D('',#23450,#19168,#19169);
#17074=AXIS2_PLACEMENT_3D('',#23454,#19171,#19172);
#17075=AXIS2_PLACEMENT_3D('',#23458,#19174,#19175);
#17076=AXIS2_PLACEMENT_3D('',#23466,#19180,#19181);
#17077=AXIS2_PLACEMENT_3D('',#23472,#19185,#19186);
#17078=AXIS2_PLACEMENT_3D('',#23480,#19191,#19192);
#17079=AXIS2_PLACEMENT_3D('',#23482,#19193,#19194);
#17080=AXIS2_PLACEMENT_3D('',#23484,#19196,#19197);
#17081=AXIS2_PLACEMENT_3D('',#23485,#19198,#19199);
#17082=AXIS2_PLACEMENT_3D('',#23487,#19200,#19201);
#17083=AXIS2_PLACEMENT_3D('',#23489,#19203,#19204);
#17084=AXIS2_PLACEMENT_3D('',#23490,#19205,#19206);
#17085=AXIS2_PLACEMENT_3D('',#23493,#19208,#19209);
#17086=AXIS2_PLACEMENT_3D('',#23494,#19210,#19211);
#17087=AXIS2_PLACEMENT_3D('',#23495,#19212,#19213);
#17088=AXIS2_PLACEMENT_3D('',#23498,#19215,#19216);
#17089=AXIS2_PLACEMENT_3D('',#23499,#19217,#19218);
#17090=AXIS2_PLACEMENT_3D('',#23500,#19219,#19220);
#17091=AXIS2_PLACEMENT_3D('',#23504,#19222,#19223);
#17092=AXIS2_PLACEMENT_3D('',#23505,#19224,#19225);
#17093=AXIS2_PLACEMENT_3D('',#23506,#19226,#19227);
#17094=AXIS2_PLACEMENT_3D('',#23508,#19229,#19230);
#17095=AXIS2_PLACEMENT_3D('',#23510,#19231,#19232);
#17096=AXIS2_PLACEMENT_3D('',#23512,#19234,#19235);
#17097=AXIS2_PLACEMENT_3D('',#23515,#19237,#19238);
#17098=AXIS2_PLACEMENT_3D('',#23516,#19239,#19240);
#17099=AXIS2_PLACEMENT_3D('',#23519,#19242,#19243);
#17100=AXIS2_PLACEMENT_3D('',#23520,#19244,#19245);
#17101=AXIS2_PLACEMENT_3D('',#23522,#19247,#19248);
#17102=AXIS2_PLACEMENT_3D('',#23528,#19252,#19253);
#17103=AXIS2_PLACEMENT_3D('',#23536,#19258,#19259);
#17104=AXIS2_PLACEMENT_3D('',#23538,#19260,#19261);
#17105=AXIS2_PLACEMENT_3D('',#23540,#19263,#19264);
#17106=AXIS2_PLACEMENT_3D('',#23541,#19265,#19266);
#17107=AXIS2_PLACEMENT_3D('',#23543,#19267,#19268);
#17108=AXIS2_PLACEMENT_3D('',#23545,#19270,#19271);
#17109=AXIS2_PLACEMENT_3D('',#23546,#19272,#19273);
#17110=AXIS2_PLACEMENT_3D('',#23549,#19275,#19276);
#17111=AXIS2_PLACEMENT_3D('',#23550,#19277,#19278);
#17112=AXIS2_PLACEMENT_3D('',#23551,#19279,#19280);
#17113=AXIS2_PLACEMENT_3D('',#23554,#19282,#19283);
#17114=AXIS2_PLACEMENT_3D('',#23555,#19284,#19285);
#17115=AXIS2_PLACEMENT_3D('',#23556,#19286,#19287);
#17116=AXIS2_PLACEMENT_3D('',#23558,#19288,#19289);
#17117=AXIS2_PLACEMENT_3D('',#23560,#19291,#19292);
#17118=AXIS2_PLACEMENT_3D('',#23562,#19293,#19294);
#17119=AXIS2_PLACEMENT_3D('',#23564,#19296,#19297);
#17120=AXIS2_PLACEMENT_3D('',#23567,#19299,#19300);
#17121=AXIS2_PLACEMENT_3D('',#23568,#19301,#19302);
#17122=AXIS2_PLACEMENT_3D('',#23571,#19304,#19305);
#17123=AXIS2_PLACEMENT_3D('',#23572,#19306,#19307);
#17124=AXIS2_PLACEMENT_3D('',#23574,#19309,#19310);
#17125=AXIS2_PLACEMENT_3D('',#23576,#19311,#19312);
#17126=AXIS2_PLACEMENT_3D('',#23578,#19314,#19315);
#17127=AXIS2_PLACEMENT_3D('',#23586,#19320,#19321);
#17128=AXIS2_PLACEMENT_3D('',#23590,#19324,#19325);
#17129=AXIS2_PLACEMENT_3D('',#23592,#19326,#19327);
#17130=AXIS2_PLACEMENT_3D('',#23594,#19328,#19329);
#17131=AXIS2_PLACEMENT_3D('',#23596,#19330,#19331);
#17132=AXIS2_PLACEMENT_3D('',#23598,#19332,#19333);
#17133=AXIS2_PLACEMENT_3D('',#23599,#19334,#19335);
#17134=AXIS2_PLACEMENT_3D('',#23602,#19337,#19338);
#17135=AXIS2_PLACEMENT_3D('',#23603,#19339,#19340);
#17136=AXIS2_PLACEMENT_3D('',#23604,#19341,#19342);
#17137=AXIS2_PLACEMENT_3D('',#23607,#19344,#19345);
#17138=AXIS2_PLACEMENT_3D('',#23608,#19346,#19347);
#17139=AXIS2_PLACEMENT_3D('',#23609,#19348,#19349);
#17140=AXIS2_PLACEMENT_3D('',#23612,#19351,#19352);
#17141=AXIS2_PLACEMENT_3D('',#23613,#19353,#19354);
#17142=AXIS2_PLACEMENT_3D('',#23614,#19355,#19356);
#17143=AXIS2_PLACEMENT_3D('',#23617,#19358,#19359);
#17144=AXIS2_PLACEMENT_3D('',#23618,#19360,#19361);
#17145=AXIS2_PLACEMENT_3D('',#23619,#19362,#19363);
#17146=AXIS2_PLACEMENT_3D('',#23622,#19365,#19366);
#17147=AXIS2_PLACEMENT_3D('',#23623,#19367,#19368);
#17148=AXIS2_PLACEMENT_3D('',#23626,#19370,#19371);
#17149=AXIS2_PLACEMENT_3D('',#23627,#19372,#19373);
#17150=AXIS2_PLACEMENT_3D('',#23630,#19375,#19376);
#17151=AXIS2_PLACEMENT_3D('',#23631,#19377,#19378);
#17152=AXIS2_PLACEMENT_3D('',#23634,#19380,#19381);
#17153=AXIS2_PLACEMENT_3D('',#23635,#19382,#19383);
#17154=AXIS2_PLACEMENT_3D('',#23638,#19385,#19386);
#17155=AXIS2_PLACEMENT_3D('',#23639,#19387,#19388);
#17156=AXIS2_PLACEMENT_3D('',#23642,#19390,#19391);
#17157=AXIS2_PLACEMENT_3D('',#23643,#19392,#19393);
#17158=AXIS2_PLACEMENT_3D('',#23645,#19395,#19396);
#17159=AXIS2_PLACEMENT_3D('',#23647,#19398,#19399);
#17160=AXIS2_PLACEMENT_3D('',#23649,#19401,#19402);
#17161=AXIS2_PLACEMENT_3D('',#23651,#19404,#19405);
#17162=AXIS2_PLACEMENT_3D('',#23653,#19407,#19408);
#17163=AXIS2_PLACEMENT_3D('',#23655,#19410,#19411);
#17164=AXIS2_PLACEMENT_3D('',#23657,#19413,#19414);
#17165=AXIS2_PLACEMENT_3D('',#23658,#19415,#19416);
#17166=AXIS2_PLACEMENT_3D('',#23660,#19418,#19419);
#18976=DIRECTION('axis',(0.,0.,1.));
#18977=DIRECTION('refdir',(1.,0.,0.));
#18978=DIRECTION('center_axis',(0.,0.,1.));
#18979=DIRECTION('ref_axis',(1.,0.,0.));
#18980=DIRECTION('center_axis',(0.,0.,1.));
#18981=DIRECTION('ref_axis',(1.,0.,0.));
#18982=DIRECTION('',(0.,0.,1.));
#18983=DIRECTION('center_axis',(0.,0.,-1.));
#18984=DIRECTION('ref_axis',(1.,0.,0.));
#18985=DIRECTION('center_axis',(0.,0.,1.));
#18986=DIRECTION('ref_axis',(1.,0.,0.));
#18987=DIRECTION('center_axis',(0.,0.,1.));
#18988=DIRECTION('ref_axis',(1.,0.,0.));
#18989=DIRECTION('',(0.,0.,1.));
#18990=DIRECTION('center_axis',(0.,0.,-1.));
#18991=DIRECTION('ref_axis',(1.,0.,0.));
#18992=DIRECTION('center_axis',(0.,0.,1.));
#18993=DIRECTION('ref_axis',(1.,0.,0.));
#18994=DIRECTION('center_axis',(0.,0.,1.));
#18995=DIRECTION('ref_axis',(1.,0.,0.));
#18996=DIRECTION('',(0.,0.,1.));
#18997=DIRECTION('center_axis',(0.,0.,-1.));
#18998=DIRECTION('ref_axis',(1.,0.,0.));
#18999=DIRECTION('center_axis',(0.,0.,1.));
#19000=DIRECTION('ref_axis',(1.,0.,0.));
#19001=DIRECTION('center_axis',(0.,0.,1.));
#19002=DIRECTION('ref_axis',(1.,0.,0.));
#19003=DIRECTION('',(0.,0.,1.));
#19004=DIRECTION('center_axis',(0.,0.,-1.));
#19005=DIRECTION('ref_axis',(1.,0.,0.));
#19006=DIRECTION('center_axis',(0.,-1.,0.));
#19007=DIRECTION('ref_axis',(1.,0.,0.));
#19008=DIRECTION('',(1.,0.,0.));
#19009=DIRECTION('',(0.,0.,1.));
#19010=DIRECTION('',(-1.,0.,0.));
#19011=DIRECTION('',(0.,0.,1.));
#19012=DIRECTION('center_axis',(1.,0.,0.));
#19013=DIRECTION('ref_axis',(0.,1.,0.));
#19014=DIRECTION('',(0.,1.,0.));
#19015=DIRECTION('',(0.,-1.,0.));
#19016=DIRECTION('',(0.,0.,1.));
#19017=DIRECTION('center_axis',(0.,1.,0.));
#19018=DIRECTION('ref_axis',(-1.,0.,0.));
#19019=DIRECTION('',(-1.,0.,0.));
#19020=DIRECTION('',(1.,0.,0.));
#19021=DIRECTION('',(0.,0.,1.));
#19022=DIRECTION('center_axis',(-1.,0.,0.));
#19023=DIRECTION('ref_axis',(0.,-1.,0.));
#19024=DIRECTION('',(0.,-1.,0.));
#19025=DIRECTION('',(0.,1.,0.));
#19026=DIRECTION('center_axis',(0.,1.,0.));
#19027=DIRECTION('ref_axis',(1.,0.,0.));
#19028=DIRECTION('center_axis',(0.,1.,0.));
#19029=DIRECTION('ref_axis',(1.,0.,0.));
#19030=DIRECTION('',(0.,1.,0.));
#19031=DIRECTION('center_axis',(0.,-1.,0.));
#19032=DIRECTION('ref_axis',(1.,0.,0.));
#19033=DIRECTION('center_axis',(0.,1.,0.));
#19034=DIRECTION('ref_axis',(1.,0.,0.));
#19035=DIRECTION('center_axis',(0.,1.,0.));
#19036=DIRECTION('ref_axis',(1.,0.,0.));
#19037=DIRECTION('center_axis',(0.,1.,0.));
#19038=DIRECTION('ref_axis',(1.,0.,0.));
#19039=DIRECTION('',(0.,1.,0.));
#19040=DIRECTION('center_axis',(0.,-1.,0.));
#19041=DIRECTION('ref_axis',(1.,0.,0.));
#19042=DIRECTION('center_axis',(0.,1.,0.));
#19043=DIRECTION('ref_axis',(1.,0.,0.));
#19044=DIRECTION('center_axis',(0.,1.,0.));
#19045=DIRECTION('ref_axis',(1.,0.,0.));
#19046=DIRECTION('center_axis',(0.,1.,0.));
#19047=DIRECTION('ref_axis',(1.,0.,0.));
#19048=DIRECTION('',(0.,1.,0.));
#19049=DIRECTION('center_axis',(0.,1.,0.));
#19050=DIRECTION('ref_axis',(1.,0.,0.));
#19051=DIRECTION('center_axis',(0.,1.,0.));
#19052=DIRECTION('ref_axis',(1.,0.,0.));
#19053=DIRECTION('center_axis',(0.,1.,0.));
#19054=DIRECTION('ref_axis',(1.,0.,0.));
#19055=DIRECTION('center_axis',(0.,1.,0.));
#19056=DIRECTION('ref_axis',(1.,0.,0.));
#19057=DIRECTION('',(0.,1.,0.));
#19058=DIRECTION('center_axis',(0.,1.,0.));
#19059=DIRECTION('ref_axis',(1.,0.,0.));
#19060=DIRECTION('center_axis',(0.,1.,0.));
#19061=DIRECTION('ref_axis',(1.,0.,0.));
#19062=DIRECTION('center_axis',(0.,1.,0.));
#19063=DIRECTION('ref_axis',(1.,0.,0.));
#19064=DIRECTION('',(1.,0.,0.));
#19065=DIRECTION('center_axis',(0.,1.,0.));
#19066=DIRECTION('ref_axis',(1.,0.,0.));
#19067=DIRECTION('',(1.,0.,0.));
#19068=DIRECTION('center_axis',(0.,1.,0.));
#19069=DIRECTION('ref_axis',(1.,0.,0.));
#19070=DIRECTION('center_axis',(0.,1.,0.));
#19071=DIRECTION('ref_axis',(1.,0.,0.));
#19072=DIRECTION('',(0.,-1.,0.));
#19073=DIRECTION('center_axis',(0.,-1.,0.));
#19074=DIRECTION('ref_axis',(1.,0.,0.));
#19075=DIRECTION('',(0.,1.,0.));
#19076=DIRECTION('center_axis',(0.,1.,0.));
#19077=DIRECTION('ref_axis',(1.,0.,0.));
#19078=DIRECTION('',(0.,1.,0.));
#19079=DIRECTION('center_axis',(0.,1.,0.));
#19080=DIRECTION('ref_axis',(1.,0.,0.));
#19081=DIRECTION('',(0.,-1.,0.));
#19082=DIRECTION('center_axis',(0.,0.,1.));
#19083=DIRECTION('ref_axis',(1.,0.,0.));
#19084=DIRECTION('',(-1.,0.,0.));
#19085=DIRECTION('',(0.,1.,0.));
#19086=DIRECTION('',(1.,0.,0.));
#19087=DIRECTION('',(0.,1.,0.));
#19088=DIRECTION('',(-1.,0.,0.));
#19089=DIRECTION('',(0.,1.,0.));
#19090=DIRECTION('',(1.,0.,0.));
#19091=DIRECTION('',(0.,1.,0.));
#19092=DIRECTION('',(-1.,0.,0.));
#19093=DIRECTION('center_axis',(0.,0.,1.));
#19094=DIRECTION('ref_axis',(1.,0.,0.));
#19095=DIRECTION('center_axis',(0.,0.,1.));
#19096=DIRECTION('ref_axis',(1.,0.,0.));
#19097=DIRECTION('center_axis',(0.,0.,1.));
#19098=DIRECTION('ref_axis',(1.,0.,0.));
#19099=DIRECTION('center_axis',(0.,0.,1.));
#19100=DIRECTION('ref_axis',(1.,0.,0.));
#19101=DIRECTION('center_axis',(0.,0.,1.));
#19102=DIRECTION('ref_axis',(1.,0.,0.));
#19103=DIRECTION('center_axis',(0.,1.,0.));
#19104=DIRECTION('ref_axis',(1.,0.,0.));
#19105=DIRECTION('',(0.,-1.,0.));
#19106=DIRECTION('center_axis',(0.,1.,0.));
#19107=DIRECTION('ref_axis',(1.,0.,0.));
#19108=DIRECTION('center_axis',(0.,1.,0.));
#19109=DIRECTION('ref_axis',(1.,0.,0.));
#19110=DIRECTION('center_axis',(0.,1.,0.));
#19111=DIRECTION('ref_axis',(1.,0.,0.));
#19112=DIRECTION('',(-1.,0.,0.));
#19113=DIRECTION('center_axis',(0.,-1.,0.));
#19114=DIRECTION('ref_axis',(1.,0.,0.));
#19115=DIRECTION('center_axis',(0.,-1.,0.));
#19116=DIRECTION('ref_axis',(1.,0.,0.));
#19117=DIRECTION('',(0.,0.,1.));
#19118=DIRECTION('',(1.,0.,0.));
#19119=DIRECTION('',(0.,0.,1.));
#19120=DIRECTION('',(1.,0.,0.));
#19121=DIRECTION('',(0.,0.,1.));
#19122=DIRECTION('',(1.,0.,0.));
#19123=DIRECTION('',(0.,0.,1.));
#19124=DIRECTION('',(1.,0.,0.));
#19125=DIRECTION('center_axis',(0.,1.,0.));
#19126=DIRECTION('ref_axis',(1.,0.,0.));
#19127=DIRECTION('',(1.,0.,0.));
#19128=DIRECTION('center_axis',(0.,1.,0.));
#19129=DIRECTION('ref_axis',(1.,0.,0.));
#19130=DIRECTION('',(1.,0.,0.));
#19131=DIRECTION('center_axis',(0.,1.,0.));
#19132=DIRECTION('ref_axis',(1.,0.,0.));
#19133=DIRECTION('center_axis',(0.,1.,0.));
#19134=DIRECTION('ref_axis',(1.,0.,0.));
#19135=DIRECTION('center_axis',(0.,1.,0.));
#19136=DIRECTION('ref_axis',(1.,0.,0.));
#19137=DIRECTION('center_axis',(0.,1.,0.));
#19138=DIRECTION('ref_axis',(1.,0.,0.));
#19139=DIRECTION('center_axis',(0.,1.,0.));
#19140=DIRECTION('ref_axis',(1.,0.,0.));
#19141=DIRECTION('',(0.,-1.,0.));
#19142=DIRECTION('center_axis',(0.,-1.,0.));
#19143=DIRECTION('ref_axis',(1.,0.,0.));
#19144=DIRECTION('center_axis',(0.,1.,0.));
#19145=DIRECTION('ref_axis',(-1.,0.,0.));
#19146=DIRECTION('',(-1.,0.,0.));
#19147=DIRECTION('center_axis',(0.,-1.,0.));
#19148=DIRECTION('ref_axis',(1.,0.,0.));
#19149=DIRECTION('',(-1.,0.,0.));
#19150=DIRECTION('center_axis',(0.,-1.,0.));
#19151=DIRECTION('ref_axis',(1.,0.,0.));
#19152=DIRECTION('',(-1.,0.,0.));
#19153=DIRECTION('',(0.,0.,1.));
#19154=DIRECTION('',(-1.,0.,0.));
#19155=DIRECTION('',(0.,0.,1.));
#19156=DIRECTION('',(-1.,0.,0.));
#19157=DIRECTION('',(0.,0.,1.));
#19158=DIRECTION('',(-1.,0.,0.));
#19159=DIRECTION('',(0.,0.,1.));
#19160=DIRECTION('center_axis',(0.,-1.,0.));
#19161=DIRECTION('ref_axis',(1.,0.,0.));
#19162=DIRECTION('center_axis',(0.,-1.,0.));
#19163=DIRECTION('ref_axis',(1.,0.,0.));
#19164=DIRECTION('center_axis',(0.,-1.,0.));
#19165=DIRECTION('ref_axis',(1.,0.,0.));
#19166=DIRECTION('center_axis',(0.,-1.,0.));
#19167=DIRECTION('ref_axis',(1.,0.,0.));
#19168=DIRECTION('center_axis',(0.,-1.,0.));
#19169=DIRECTION('ref_axis',(1.,0.,0.));
#19170=DIRECTION('',(1.,0.,0.));
#19171=DIRECTION('center_axis',(0.,-1.,0.));
#19172=DIRECTION('ref_axis',(1.,0.,0.));
#19173=DIRECTION('',(1.,0.,0.));
#19174=DIRECTION('center_axis',(0.,-1.,0.));
#19175=DIRECTION('ref_axis',(1.,0.,0.));
#19176=DIRECTION('',(1.,0.,0.));
#19177=DIRECTION('',(0.,0.,1.));
#19178=DIRECTION('',(1.,0.,0.));
#19179=DIRECTION('',(0.,0.,1.));
#19180=DIRECTION('center_axis',(0.,0.,1.));
#19181=DIRECTION('ref_axis',(1.,0.,0.));
#19182=DIRECTION('',(0.,1.,0.));
#19183=DIRECTION('',(-1.,0.,0.));
#19184=DIRECTION('',(0.,1.,0.));
#19185=DIRECTION('center_axis',(0.,0.,1.));
#19186=DIRECTION('ref_axis',(1.,0.,0.));
#19187=DIRECTION('',(-1.,0.,0.));
#19188=DIRECTION('',(0.,1.,0.));
#19189=DIRECTION('',(1.,0.,0.));
#19190=DIRECTION('',(0.,1.,0.));
#19191=DIRECTION('center_axis',(0.,1.,0.));
#19192=DIRECTION('ref_axis',(1.,0.,0.));
#19193=DIRECTION('center_axis',(0.,1.,0.));
#19194=DIRECTION('ref_axis',(1.,0.,0.));
#19195=DIRECTION('',(0.,1.,0.));
#19196=DIRECTION('center_axis',(0.,1.,0.));
#19197=DIRECTION('ref_axis',(1.,0.,0.));
#19198=DIRECTION('center_axis',(0.,1.,0.));
#19199=DIRECTION('ref_axis',(1.,0.,0.));
#19200=DIRECTION('center_axis',(0.,1.,0.));
#19201=DIRECTION('ref_axis',(1.,0.,0.));
#19202=DIRECTION('',(0.,1.,0.));
#19203=DIRECTION('center_axis',(0.,1.,0.));
#19204=DIRECTION('ref_axis',(1.,0.,0.));
#19205=DIRECTION('center_axis',(0.,1.,0.));
#19206=DIRECTION('ref_axis',(1.,0.,0.));
#19207=DIRECTION('',(0.,1.,0.));
#19208=DIRECTION('center_axis',(0.,1.,0.));
#19209=DIRECTION('ref_axis',(1.,0.,0.));
#19210=DIRECTION('center_axis',(0.,1.,0.));
#19211=DIRECTION('ref_axis',(1.,0.,0.));
#19212=DIRECTION('center_axis',(0.,1.,0.));
#19213=DIRECTION('ref_axis',(1.,0.,0.));
#19214=DIRECTION('',(0.,1.,0.));
#19215=DIRECTION('center_axis',(0.,1.,0.));
#19216=DIRECTION('ref_axis',(1.,0.,0.));
#19217=DIRECTION('center_axis',(0.,1.,0.));
#19218=DIRECTION('ref_axis',(1.,0.,0.));
#19219=DIRECTION('center_axis',(0.,1.,0.));
#19220=DIRECTION('ref_axis',(1.,0.,0.));
#19221=DIRECTION('',(1.,0.,0.));
#19222=DIRECTION('center_axis',(0.,1.,0.));
#19223=DIRECTION('ref_axis',(1.,0.,0.));
#19224=DIRECTION('center_axis',(0.,1.,0.));
#19225=DIRECTION('ref_axis',(1.,0.,0.));
#19226=DIRECTION('center_axis',(0.,1.,0.));
#19227=DIRECTION('ref_axis',(1.,0.,0.));
#19228=DIRECTION('',(0.,-1.,0.));
#19229=DIRECTION('center_axis',(0.,1.,0.));
#19230=DIRECTION('ref_axis',(1.,0.,0.));
#19231=DIRECTION('center_axis',(0.,1.,0.));
#19232=DIRECTION('ref_axis',(1.,0.,0.));
#19233=DIRECTION('',(0.,-1.,0.));
#19234=DIRECTION('center_axis',(0.,1.,0.));
#19235=DIRECTION('ref_axis',(1.,0.,0.));
#19236=DIRECTION('',(0.,-1.,0.));
#19237=DIRECTION('center_axis',(0.,1.,0.));
#19238=DIRECTION('ref_axis',(1.,0.,0.));
#19239=DIRECTION('center_axis',(0.,1.,0.));
#19240=DIRECTION('ref_axis',(1.,0.,0.));
#19241=DIRECTION('',(-1.,0.,0.));
#19242=DIRECTION('center_axis',(0.,-1.,0.));
#19243=DIRECTION('ref_axis',(1.,0.,0.));
#19244=DIRECTION('center_axis',(0.,1.,0.));
#19245=DIRECTION('ref_axis',(1.,0.,0.));
#19246=DIRECTION('',(0.,-1.,0.));
#19247=DIRECTION('center_axis',(0.,0.,1.));
#19248=DIRECTION('ref_axis',(1.,0.,0.));
#19249=DIRECTION('',(0.,1.,0.));
#19250=DIRECTION('',(-1.,0.,0.));
#19251=DIRECTION('',(0.,1.,0.));
#19252=DIRECTION('center_axis',(0.,0.,1.));
#19253=DIRECTION('ref_axis',(1.,0.,0.));
#19254=DIRECTION('',(-1.,0.,0.));
#19255=DIRECTION('',(0.,1.,0.));
#19256=DIRECTION('',(1.,0.,0.));
#19257=DIRECTION('',(0.,1.,0.));
#19258=DIRECTION('center_axis',(0.,1.,0.));
#19259=DIRECTION('ref_axis',(1.,0.,0.));
#19260=DIRECTION('center_axis',(0.,1.,0.));
#19261=DIRECTION('ref_axis',(1.,0.,0.));
#19262=DIRECTION('',(0.,1.,0.));
#19263=DIRECTION('center_axis',(0.,1.,0.));
#19264=DIRECTION('ref_axis',(1.,0.,0.));
#19265=DIRECTION('center_axis',(0.,1.,0.));
#19266=DIRECTION('ref_axis',(1.,0.,0.));
#19267=DIRECTION('center_axis',(0.,1.,0.));
#19268=DIRECTION('ref_axis',(1.,0.,0.));
#19269=DIRECTION('',(0.,1.,0.));
#19270=DIRECTION('center_axis',(0.,1.,0.));
#19271=DIRECTION('ref_axis',(1.,0.,0.));
#19272=DIRECTION('center_axis',(0.,1.,0.));
#19273=DIRECTION('ref_axis',(1.,0.,0.));
#19274=DIRECTION('',(0.,1.,0.));
#19275=DIRECTION('center_axis',(0.,1.,0.));
#19276=DIRECTION('ref_axis',(1.,0.,0.));
#19277=DIRECTION('center_axis',(0.,1.,0.));
#19278=DIRECTION('ref_axis',(1.,0.,0.));
#19279=DIRECTION('center_axis',(0.,1.,0.));
#19280=DIRECTION('ref_axis',(1.,0.,0.));
#19281=DIRECTION('',(0.,1.,0.));
#19282=DIRECTION('center_axis',(0.,1.,0.));
#19283=DIRECTION('ref_axis',(1.,0.,0.));
#19284=DIRECTION('center_axis',(0.,1.,0.));
#19285=DIRECTION('ref_axis',(1.,0.,0.));
#19286=DIRECTION('center_axis',(0.,1.,0.));
#19287=DIRECTION('ref_axis',(1.,0.,0.));
#19288=DIRECTION('center_axis',(0.,1.,0.));
#19289=DIRECTION('ref_axis',(1.,0.,0.));
#19290=DIRECTION('',(0.,-1.,0.));
#19291=DIRECTION('center_axis',(0.,1.,0.));
#19292=DIRECTION('ref_axis',(1.,0.,0.));
#19293=DIRECTION('center_axis',(0.,1.,0.));
#19294=DIRECTION('ref_axis',(1.,0.,0.));
#19295=DIRECTION('',(1.,0.,0.));
#19296=DIRECTION('center_axis',(0.,1.,0.));
#19297=DIRECTION('ref_axis',(1.,0.,0.));
#19298=DIRECTION('',(0.,-1.,0.));
#19299=DIRECTION('center_axis',(0.,1.,0.));
#19300=DIRECTION('ref_axis',(1.,0.,0.));
#19301=DIRECTION('center_axis',(0.,1.,0.));
#19302=DIRECTION('ref_axis',(1.,0.,0.));
#19303=DIRECTION('',(-1.,0.,0.));
#19304=DIRECTION('center_axis',(0.,-1.,0.));
#19305=DIRECTION('ref_axis',(1.,0.,0.));
#19306=DIRECTION('center_axis',(0.,1.,0.));
#19307=DIRECTION('ref_axis',(1.,0.,0.));
#19308=DIRECTION('',(0.,-1.,0.));
#19309=DIRECTION('center_axis',(0.,1.,0.));
#19310=DIRECTION('ref_axis',(1.,0.,0.));
#19311=DIRECTION('center_axis',(0.,1.,0.));
#19312=DIRECTION('ref_axis',(1.,0.,0.));
#19313=DIRECTION('',(0.,-1.,0.));
#19314=DIRECTION('center_axis',(0.,1.,0.));
#19315=DIRECTION('ref_axis',(-1.,0.,0.));
#19316=DIRECTION('',(0.,0.,1.));
#19317=DIRECTION('',(-1.,0.,0.));
#19318=DIRECTION('',(0.,0.,1.));
#19319=DIRECTION('',(-1.,0.,0.));
#19320=DIRECTION('center_axis',(0.,0.,1.));
#19321=DIRECTION('ref_axis',(1.,0.,0.));
#19322=DIRECTION('',(0.,-1.,0.));
#19323=DIRECTION('',(0.,-1.,0.));
#19324=DIRECTION('center_axis',(0.,0.,1.));
#19325=DIRECTION('ref_axis',(1.,0.,0.));
#19326=DIRECTION('center_axis',(0.,0.,1.));
#19327=DIRECTION('ref_axis',(1.,0.,0.));
#19328=DIRECTION('center_axis',(0.,0.,1.));
#19329=DIRECTION('ref_axis',(1.,0.,0.));
#19330=DIRECTION('center_axis',(0.,0.,1.));
#19331=DIRECTION('ref_axis',(1.,0.,0.));
#19332=DIRECTION('center_axis',(0.,0.,1.));
#19333=DIRECTION('ref_axis',(1.,0.,0.));
#19334=DIRECTION('center_axis',(0.,0.,1.));
#19335=DIRECTION('ref_axis',(1.,0.,0.));
#19336=DIRECTION('',(0.,0.,1.));
#19337=DIRECTION('center_axis',(0.,0.,1.));
#19338=DIRECTION('ref_axis',(1.,0.,0.));
#19339=DIRECTION('center_axis',(0.,0.,1.));
#19340=DIRECTION('ref_axis',(1.,0.,0.));
#19341=DIRECTION('center_axis',(0.,0.,1.));
#19342=DIRECTION('ref_axis',(1.,0.,0.));
#19343=DIRECTION('',(0.,0.,1.));
#19344=DIRECTION('center_axis',(0.,0.,1.));
#19345=DIRECTION('ref_axis',(1.,0.,0.));
#19346=DIRECTION('center_axis',(0.,0.,1.));
#19347=DIRECTION('ref_axis',(1.,0.,0.));
#19348=DIRECTION('center_axis',(0.,0.,1.));
#19349=DIRECTION('ref_axis',(1.,0.,0.));
#19350=DIRECTION('',(0.,0.,1.));
#19351=DIRECTION('center_axis',(0.,0.,1.));
#19352=DIRECTION('ref_axis',(1.,0.,0.));
#19353=DIRECTION('center_axis',(0.,0.,1.));
#19354=DIRECTION('ref_axis',(1.,0.,0.));
#19355=DIRECTION('center_axis',(0.,0.,1.));
#19356=DIRECTION('ref_axis',(1.,0.,0.));
#19357=DIRECTION('',(0.,0.,1.));
#19358=DIRECTION('center_axis',(0.,0.,1.));
#19359=DIRECTION('ref_axis',(1.,0.,0.));
#19360=DIRECTION('center_axis',(0.,0.,1.));
#19361=DIRECTION('ref_axis',(1.,0.,0.));
#19362=DIRECTION('center_axis',(0.,0.,1.));
#19363=DIRECTION('ref_axis',(1.,0.,0.));
#19364=DIRECTION('',(0.,0.,1.));
#19365=DIRECTION('center_axis',(0.,0.,-1.));
#19366=DIRECTION('ref_axis',(1.,0.,0.));
#19367=DIRECTION('center_axis',(0.,0.,1.));
#19368=DIRECTION('ref_axis',(1.,0.,0.));
#19369=DIRECTION('',(0.,0.,1.));
#19370=DIRECTION('center_axis',(0.,0.,-1.));
#19371=DIRECTION('ref_axis',(1.,0.,0.));
#19372=DIRECTION('center_axis',(0.,0.,1.));
#19373=DIRECTION('ref_axis',(1.,0.,0.));
#19374=DIRECTION('',(0.,0.,1.));
#19375=DIRECTION('center_axis',(0.,0.,-1.));
#19376=DIRECTION('ref_axis',(1.,0.,0.));
#19377=DIRECTION('center_axis',(0.,0.,1.));
#19378=DIRECTION('ref_axis',(1.,0.,0.));
#19379=DIRECTION('',(0.,0.,1.));
#19380=DIRECTION('center_axis',(0.,0.,-1.));
#19381=DIRECTION('ref_axis',(1.,0.,0.));
#19382=DIRECTION('center_axis',(0.,0.,1.));
#19383=DIRECTION('ref_axis',(1.,0.,0.));
#19384=DIRECTION('',(0.,0.,1.));
#19385=DIRECTION('center_axis',(0.,0.,-1.));
#19386=DIRECTION('ref_axis',(1.,0.,0.));
#19387=DIRECTION('center_axis',(0.,0.,1.));
#19388=DIRECTION('ref_axis',(1.,0.,0.));
#19389=DIRECTION('',(0.,0.,1.));
#19390=DIRECTION('center_axis',(0.,0.,-1.));
#19391=DIRECTION('ref_axis',(1.,0.,0.));
#19392=DIRECTION('center_axis',(1.,0.,0.));
#19393=DIRECTION('ref_axis',(0.,1.,0.));
#19394=DIRECTION('',(0.,1.,0.));
#19395=DIRECTION('center_axis',(0.,0.,1.));
#19396=DIRECTION('ref_axis',(1.,0.,0.));
#19397=DIRECTION('',(0.,1.,0.));
#19398=DIRECTION('center_axis',(-1.,0.,0.));
#19399=DIRECTION('ref_axis',(0.,-1.,0.));
#19400=DIRECTION('',(0.,-1.,0.));
#19401=DIRECTION('center_axis',(0.,0.,1.));
#19402=DIRECTION('ref_axis',(1.,0.,0.));
#19403=DIRECTION('',(0.,-1.,0.));
#19404=DIRECTION('center_axis',(-1.,0.,0.));
#19405=DIRECTION('ref_axis',(0.,-1.,0.));
#19406=DIRECTION('',(0.,-1.,0.));
#19407=DIRECTION('center_axis',(1.,0.,0.));
#19408=DIRECTION('ref_axis',(0.,1.,0.));
#19409=DIRECTION('',(0.,1.,0.));
#19410=DIRECTION('center_axis',(-1.,0.,0.));
#19411=DIRECTION('ref_axis',(0.,-1.,0.));
#19412=DIRECTION('',(0.,-1.,0.));
#19413=DIRECTION('center_axis',(0.,0.,1.));
#19414=DIRECTION('ref_axis',(1.,0.,0.));
#19415=DIRECTION('center_axis',(1.,0.,0.));
#19416=DIRECTION('ref_axis',(0.,1.,0.));
#19417=DIRECTION('',(0.,1.,0.));
#19418=DIRECTION('center_axis',(0.,0.,1.));
#19419=DIRECTION('ref_axis',(1.,0.,0.));
#23246=CARTESIAN_POINT('',(0.,0.,0.));
#23247=CARTESIAN_POINT('Origin',(14.5,-3.5,14.8));
#23248=CARTESIAN_POINT('',(14.335,-3.5,15.));
#23249=CARTESIAN_POINT('Origin',(14.5,-3.5,15.));
#23250=CARTESIAN_POINT('',(14.335,-3.5,16.));
#23251=CARTESIAN_POINT('',(14.335,-3.5,14.8));
#23252=CARTESIAN_POINT('Origin',(14.5,-3.5,16.));
#23253=CARTESIAN_POINT('Origin',(1.5,3.5,14.8));
#23254=CARTESIAN_POINT('',(1.335,3.5,15.));
#23255=CARTESIAN_POINT('Origin',(1.5,3.5,15.));
#23256=CARTESIAN_POINT('',(1.335,3.5,16.));
#23257=CARTESIAN_POINT('',(1.335,3.5,14.8));
#23258=CARTESIAN_POINT('Origin',(1.5,3.5,16.));
#23259=CARTESIAN_POINT('Origin',(1.5,-3.5,14.8));
#23260=CARTESIAN_POINT('',(1.335,-3.5,15.));
#23261=CARTESIAN_POINT('Origin',(1.5,-3.5,15.));
#23262=CARTESIAN_POINT('',(1.335,-3.5,16.));
#23263=CARTESIAN_POINT('',(1.335,-3.5,14.8));
#23264=CARTESIAN_POINT('Origin',(1.5,-3.5,16.));
#23265=CARTESIAN_POINT('Origin',(14.5,3.5,14.8));
#23266=CARTESIAN_POINT('',(14.335,3.5,15.));
#23267=CARTESIAN_POINT('Origin',(14.5,3.5,15.));
#23268=CARTESIAN_POINT('',(14.335,3.5,16.));
#23269=CARTESIAN_POINT('',(14.335,3.5,14.8));
#23270=CARTESIAN_POINT('Origin',(14.5,3.5,16.));
#23271=CARTESIAN_POINT('Origin',(2.,-3.,14.9));
#23272=CARTESIAN_POINT('',(2.,-3.,15.));
#23273=CARTESIAN_POINT('',(14.,-3.,15.));
#23274=CARTESIAN_POINT('',(4.3,-3.,15.));
#23275=CARTESIAN_POINT('',(2.,-3.,16.));
#23276=CARTESIAN_POINT('',(2.,-3.,14.9));
#23277=CARTESIAN_POINT('',(14.,-3.,16.));
#23278=CARTESIAN_POINT('',(4.25,-3.,16.));
#23279=CARTESIAN_POINT('',(14.,-3.,14.9));
#23280=CARTESIAN_POINT('Origin',(14.,-3.,14.9));
#23281=CARTESIAN_POINT('',(14.,3.,15.));
#23282=CARTESIAN_POINT('',(14.,-1.5,15.));
#23283=CARTESIAN_POINT('',(14.,3.,16.));
#23284=CARTESIAN_POINT('',(14.,-1.5,16.));
#23285=CARTESIAN_POINT('',(14.,3.,14.9));
#23286=CARTESIAN_POINT('Origin',(14.,3.,14.9));
#23287=CARTESIAN_POINT('',(2.,3.,15.));
#23288=CARTESIAN_POINT('',(10.3,3.,15.));
#23289=CARTESIAN_POINT('',(2.,3.,16.));
#23290=CARTESIAN_POINT('',(10.25,3.,16.));
#23291=CARTESIAN_POINT('',(2.,3.,14.9));
#23292=CARTESIAN_POINT('Origin',(2.,3.,14.9));
#23293=CARTESIAN_POINT('',(2.,1.5,15.));
#23294=CARTESIAN_POINT('',(2.,1.5,16.));
#23295=CARTESIAN_POINT('Origin',(10.161522368915,6.1,11.838477631085));
#23296=CARTESIAN_POINT('',(9.99652236891498,6.1,11.838477631085));
#23297=CARTESIAN_POINT('Origin',(10.161522368915,6.1,11.838477631085));
#23298=CARTESIAN_POINT('',(9.99652236891498,7.5,11.838477631085));
#23299=CARTESIAN_POINT('',(9.99652236891498,6.1,11.838477631085));
#23300=CARTESIAN_POINT('Origin',(10.161522368915,7.5,11.838477631085));
#23301=CARTESIAN_POINT('Origin',(10.161522368915,6.1,11.838477631085));
#23302=CARTESIAN_POINT('Origin',(13.838477631085,6.1,11.838477631085));
#23303=CARTESIAN_POINT('',(13.673477631085,6.1,11.838477631085));
#23304=CARTESIAN_POINT('Origin',(13.838477631085,6.1,11.838477631085));
#23305=CARTESIAN_POINT('',(13.673477631085,7.5,11.838477631085));
#23306=CARTESIAN_POINT('',(13.673477631085,6.1,11.838477631085));
#23307=CARTESIAN_POINT('Origin',(13.838477631085,7.5,11.838477631085));
#23308=CARTESIAN_POINT('Origin',(13.838477631085,6.1,11.838477631085));
#23309=CARTESIAN_POINT('Origin',(10.161522368915,-7.6,11.838477631085));
#23310=CARTESIAN_POINT('',(9.99652236891498,-7.5,11.838477631085));
#23311=CARTESIAN_POINT('Origin',(10.161522368915,-7.5,11.838477631085));
#23312=CARTESIAN_POINT('',(9.99652236891498,-6.1,11.838477631085));
#23313=CARTESIAN_POINT('',(9.99652236891498,-7.6,11.838477631085));
#23314=CARTESIAN_POINT('Origin',(10.161522368915,-6.1,11.838477631085));
#23315=CARTESIAN_POINT('Origin',(10.161522368915,-6.1,11.838477631085));
#23316=CARTESIAN_POINT('Origin',(13.838477631085,-7.6,11.838477631085));
#23317=CARTESIAN_POINT('',(13.673477631085,-7.5,11.838477631085));
#23318=CARTESIAN_POINT('Origin',(13.838477631085,-7.5,11.838477631085));
#23319=CARTESIAN_POINT('',(13.673477631085,-6.1,11.838477631085));
#23320=CARTESIAN_POINT('',(13.673477631085,-7.6,11.838477631085));
#23321=CARTESIAN_POINT('Origin',(13.838477631085,-6.1,11.838477631085));
#23322=CARTESIAN_POINT('Origin',(13.838477631085,-6.1,11.838477631085));
#23323=CARTESIAN_POINT('Origin',(12.,5.3,10.));
#23324=CARTESIAN_POINT('',(9.65,5.3,10.));
#23325=CARTESIAN_POINT('',(10.1,5.3,10.));
#23326=CARTESIAN_POINT('',(9.25,5.3,10.));
#23327=CARTESIAN_POINT('',(14.35,5.3,10.));
#23328=CARTESIAN_POINT('Origin',(12.,5.3,10.));
#23329=CARTESIAN_POINT('',(13.9,5.3,10.));
#23330=CARTESIAN_POINT('',(9.25,5.3,10.));
#23331=CARTESIAN_POINT('Origin',(12.,5.3,10.));
#23332=CARTESIAN_POINT('Origin',(12.,5.3,10.));
#23333=CARTESIAN_POINT('',(9.65,7.5,10.));
#23334=CARTESIAN_POINT('',(9.65,5.3,10.));
#23335=CARTESIAN_POINT('',(14.35,7.5,10.));
#23336=CARTESIAN_POINT('Origin',(12.,7.5,10.));
#23337=CARTESIAN_POINT('',(14.35,5.3,10.));
#23338=CARTESIAN_POINT('Origin',(12.,-7.6,10.));
#23339=CARTESIAN_POINT('',(13.9,5.,10.));
#23340=CARTESIAN_POINT('',(13.9,-7.6,10.));
#23341=CARTESIAN_POINT('',(10.1,5.,10.));
#23342=CARTESIAN_POINT('Origin',(12.,5.,10.));
#23343=CARTESIAN_POINT('',(10.1,-7.6,10.));
#23344=CARTESIAN_POINT('Origin',(6.5,0.,10.));
#23345=CARTESIAN_POINT('',(18.5,7.5,10.));
#23346=CARTESIAN_POINT('',(18.5,7.5,10.));
#23347=CARTESIAN_POINT('',(18.5,-7.5,10.));
#23348=CARTESIAN_POINT('',(18.5,-7.5,10.));
#23349=CARTESIAN_POINT('',(14.35,-7.5,10.));
#23350=CARTESIAN_POINT('',(-5.5,-7.5,10.));
#23351=CARTESIAN_POINT('',(14.35,-5.3,10.));
#23352=CARTESIAN_POINT('',(14.35,-7.6,10.));
#23353=CARTESIAN_POINT('',(13.9,-5.3,10.));
#23354=CARTESIAN_POINT('',(9.25,-5.3,10.));
#23355=CARTESIAN_POINT('',(13.9,-5.,10.));
#23356=CARTESIAN_POINT('',(13.9,-7.6,10.));
#23357=CARTESIAN_POINT('',(16.4,-5.,10.));
#23358=CARTESIAN_POINT('',(1.65,-5.,10.));
#23359=CARTESIAN_POINT('',(16.4,5.,10.));
#23360=CARTESIAN_POINT('',(16.4,-2.5,10.));
#23361=CARTESIAN_POINT('',(11.45,5.,10.));
#23362=CARTESIAN_POINT('',(17.6,3.,10.));
#23363=CARTESIAN_POINT('Origin',(17.75,3.,10.));
#23364=CARTESIAN_POINT('',(17.42,-4.04133443718624E-17,10.));
#23365=CARTESIAN_POINT('Origin',(17.75,0.,10.));
#23366=CARTESIAN_POINT('',(17.42,-6.,10.));
#23367=CARTESIAN_POINT('Origin',(17.75,-6.,10.));
#23368=CARTESIAN_POINT('',(17.42,6.,10.));
#23369=CARTESIAN_POINT('Origin',(17.75,6.,10.));
#23370=CARTESIAN_POINT('',(17.6,-3.,10.));
#23371=CARTESIAN_POINT('Origin',(17.75,-3.,10.));
#23372=CARTESIAN_POINT('Origin',(12.,-7.6,10.));
#23373=CARTESIAN_POINT('',(9.65,-5.3,10.));
#23374=CARTESIAN_POINT('',(9.65,-7.5,10.));
#23375=CARTESIAN_POINT('',(9.65,-7.6,10.));
#23376=CARTESIAN_POINT('Origin',(12.,-5.3,10.));
#23377=CARTESIAN_POINT('Origin',(12.,-7.5,10.));
#23378=CARTESIAN_POINT('Origin',(12.,-5.3,10.));
#23379=CARTESIAN_POINT('',(10.1,-5.3,10.));
#23380=CARTESIAN_POINT('',(9.25,-5.3,10.));
#23381=CARTESIAN_POINT('Origin',(12.,-5.3,10.));
#23382=CARTESIAN_POINT('Origin',(-4.,-7.5,10.));
#23383=CARTESIAN_POINT('',(18.5,-7.5,10.8));
#23384=CARTESIAN_POINT('',(18.5,-7.5,10.));
#23385=CARTESIAN_POINT('',(17.,-7.5,10.8));
#23386=CARTESIAN_POINT('',(17.,-7.5,10.8));
#23387=CARTESIAN_POINT('',(17.,-7.5,16.));
#23388=CARTESIAN_POINT('',(17.,-7.5,10.));
#23389=CARTESIAN_POINT('',(-4.,-7.5,16.));
#23390=CARTESIAN_POINT('',(-4.,-7.5,16.));
#23391=CARTESIAN_POINT('',(-4.,-7.5,10.8));
#23392=CARTESIAN_POINT('',(-4.,-7.5,10.));
#23393=CARTESIAN_POINT('',(-5.5,-7.5,10.8));
#23394=CARTESIAN_POINT('',(-5.5,-7.5,10.8));
#23395=CARTESIAN_POINT('',(-5.5,-7.5,10.));
#23396=CARTESIAN_POINT('',(-5.5,-7.5,10.));
#23397=CARTESIAN_POINT('',(-1.6,-7.5,10.));
#23398=CARTESIAN_POINT('',(-5.5,-7.5,10.));
#23399=CARTESIAN_POINT('',(1.6,-7.5,10.));
#23400=CARTESIAN_POINT('Origin',(0.,-7.5,10.));
#23401=CARTESIAN_POINT('',(3.65,-7.5,10.));
#23402=CARTESIAN_POINT('',(-5.5,-7.5,10.));
#23403=CARTESIAN_POINT('',(8.35,-7.5,10.));
#23404=CARTESIAN_POINT('Origin',(6.,-7.5,10.));
#23405=CARTESIAN_POINT('',(-5.5,-7.5,10.));
#23406=CARTESIAN_POINT('',(-1.57921356237309,-7.5,11.4142135623731));
#23407=CARTESIAN_POINT('Origin',(-1.41421356237309,-7.5,11.4142135623731));
#23408=CARTESIAN_POINT('',(1.2492135623731,-7.5,11.4142135623731));
#23409=CARTESIAN_POINT('Origin',(1.4142135623731,-7.5,11.4142135623731));
#23410=CARTESIAN_POINT('',(7.67347763108502,-7.5,11.838477631085));
#23411=CARTESIAN_POINT('Origin',(7.83847763108502,-7.5,11.838477631085));
#23412=CARTESIAN_POINT('',(3.99652236891498,-7.5,11.838477631085));
#23413=CARTESIAN_POINT('Origin',(4.16152236891498,-7.5,11.838477631085));
#23414=CARTESIAN_POINT('Origin',(12.,-7.6,10.));
#23415=CARTESIAN_POINT('',(10.1,-5.,10.));
#23416=CARTESIAN_POINT('',(10.1,-7.6,10.));
#23417=CARTESIAN_POINT('Origin',(12.,-5.,10.));
#23418=CARTESIAN_POINT('Origin',(17.,7.5,10.));
#23419=CARTESIAN_POINT('',(8.35,7.5,10.));
#23420=CARTESIAN_POINT('',(18.5,7.5,10.));
#23421=CARTESIAN_POINT('',(3.65,7.5,10.));
#23422=CARTESIAN_POINT('Origin',(6.,7.5,10.));
#23423=CARTESIAN_POINT('',(1.6,7.5,10.));
#23424=CARTESIAN_POINT('',(18.5,7.5,10.));
#23425=CARTESIAN_POINT('',(-1.6,7.5,10.));
#23426=CARTESIAN_POINT('Origin',(0.,7.5,10.));
#23427=CARTESIAN_POINT('',(-5.5,7.5,10.));
#23428=CARTESIAN_POINT('',(18.5,7.5,10.));
#23429=CARTESIAN_POINT('',(-5.5,7.5,10.8));
#23430=CARTESIAN_POINT('',(-5.5,7.5,10.));
#23431=CARTESIAN_POINT('',(-4.,7.5,10.8));
#23432=CARTESIAN_POINT('',(-4.,7.5,10.8));
#23433=CARTESIAN_POINT('',(-4.,7.5,16.));
#23434=CARTESIAN_POINT('',(-4.,7.5,10.));
#23435=CARTESIAN_POINT('',(17.,7.5,16.));
#23436=CARTESIAN_POINT('',(17.,7.5,16.));
#23437=CARTESIAN_POINT('',(17.,7.5,10.8));
#23438=CARTESIAN_POINT('',(17.,7.5,10.));
#23439=CARTESIAN_POINT('',(18.5,7.5,10.8));
#23440=CARTESIAN_POINT('',(18.5,7.5,10.8));
#23441=CARTESIAN_POINT('',(18.5,7.5,10.));
#23442=CARTESIAN_POINT('',(-1.57921356237309,7.5,11.4142135623731));
#23443=CARTESIAN_POINT('Origin',(-1.41421356237309,7.5,11.4142135623731));
#23444=CARTESIAN_POINT('',(1.2492135623731,7.5,11.4142135623731));
#23445=CARTESIAN_POINT('Origin',(1.4142135623731,7.5,11.4142135623731));
#23446=CARTESIAN_POINT('',(7.67347763108502,7.5,11.838477631085));
#23447=CARTESIAN_POINT('Origin',(7.83847763108502,7.5,11.838477631085));
#23448=CARTESIAN_POINT('',(3.99652236891498,7.5,11.838477631085));
#23449=CARTESIAN_POINT('Origin',(4.16152236891498,7.5,11.838477631085));
#23450=CARTESIAN_POINT('Origin',(-3.2,-5.,9.9));
#23451=CARTESIAN_POINT('',(7.9,-5.,10.));
#23452=CARTESIAN_POINT('',(1.65,-5.,10.));
#23453=CARTESIAN_POINT('',(4.1,-5.,10.));
#23454=CARTESIAN_POINT('Origin',(6.,-5.,10.));
#23455=CARTESIAN_POINT('',(1.2,-5.,10.));
#23456=CARTESIAN_POINT('',(1.65,-5.,10.));
#23457=CARTESIAN_POINT('',(-1.2,-5.,10.));
#23458=CARTESIAN_POINT('Origin',(0.,-5.,10.));
#23459=CARTESIAN_POINT('',(-3.2,-5.,10.));
#23460=CARTESIAN_POINT('',(1.65,-5.,10.));
#23461=CARTESIAN_POINT('',(-3.2,-5.,15.));
#23462=CARTESIAN_POINT('',(-3.2,-5.,9.9));
#23463=CARTESIAN_POINT('',(16.4,-5.,15.));
#23464=CARTESIAN_POINT('',(-3.2,-5.,15.));
#23465=CARTESIAN_POINT('',(16.4,-5.,9.9));
#23466=CARTESIAN_POINT('Origin',(6.5,0.,10.));
#23467=CARTESIAN_POINT('',(8.35,-5.3,10.));
#23468=CARTESIAN_POINT('',(8.35,-7.6,10.));
#23469=CARTESIAN_POINT('',(7.9,-5.3,10.));
#23470=CARTESIAN_POINT('',(6.25,-5.3,10.));
#23471=CARTESIAN_POINT('',(7.9,-7.6,10.));
#23472=CARTESIAN_POINT('Origin',(6.5,0.,10.));
#23473=CARTESIAN_POINT('',(7.9,5.,10.));
#23474=CARTESIAN_POINT('',(11.45,5.,10.));
#23475=CARTESIAN_POINT('',(7.9,5.3,10.));
#23476=CARTESIAN_POINT('',(7.9,-7.6,10.));
#23477=CARTESIAN_POINT('',(8.35,5.3,10.));
#23478=CARTESIAN_POINT('',(6.25,5.3,10.));
#23479=CARTESIAN_POINT('',(8.35,5.3,10.));
#23480=CARTESIAN_POINT('Origin',(4.16152236891498,6.1,11.838477631085));
#23481=CARTESIAN_POINT('',(3.99652236891498,6.1,11.838477631085));
#23482=CARTESIAN_POINT('Origin',(4.16152236891498,6.1,11.838477631085));
#23483=CARTESIAN_POINT('',(3.99652236891498,6.1,11.838477631085));
#23484=CARTESIAN_POINT('Origin',(4.16152236891498,6.1,11.838477631085));
#23485=CARTESIAN_POINT('Origin',(7.83847763108502,6.1,11.838477631085));
#23486=CARTESIAN_POINT('',(7.67347763108502,6.1,11.838477631085));
#23487=CARTESIAN_POINT('Origin',(7.83847763108502,6.1,11.838477631085));
#23488=CARTESIAN_POINT('',(7.67347763108502,6.1,11.838477631085));
#23489=CARTESIAN_POINT('Origin',(7.83847763108502,6.1,11.838477631085));
#23490=CARTESIAN_POINT('Origin',(4.16152236891498,-7.6,11.838477631085));
#23491=CARTESIAN_POINT('',(3.99652236891498,-6.1,11.838477631085));
#23492=CARTESIAN_POINT('',(3.99652236891498,-7.6,11.838477631085));
#23493=CARTESIAN_POINT('Origin',(4.16152236891498,-6.1,11.838477631085));
#23494=CARTESIAN_POINT('Origin',(4.16152236891498,-6.1,11.838477631085));
#23495=CARTESIAN_POINT('Origin',(7.83847763108502,-7.6,11.838477631085));
#23496=CARTESIAN_POINT('',(7.67347763108502,-6.1,11.838477631085));
#23497=CARTESIAN_POINT('',(7.67347763108502,-7.6,11.838477631085));
#23498=CARTESIAN_POINT('Origin',(7.83847763108502,-6.1,11.838477631085));
#23499=CARTESIAN_POINT('Origin',(7.83847763108502,-6.1,11.838477631085));
#23500=CARTESIAN_POINT('Origin',(6.,5.3,10.));
#23501=CARTESIAN_POINT('',(3.65,5.3,10.));
#23502=CARTESIAN_POINT('',(4.1,5.3,10.));
#23503=CARTESIAN_POINT('',(6.25,5.3,10.));
#23504=CARTESIAN_POINT('Origin',(6.,5.3,10.));
#23505=CARTESIAN_POINT('Origin',(6.,5.3,10.));
#23506=CARTESIAN_POINT('Origin',(6.,5.3,10.));
#23507=CARTESIAN_POINT('',(3.65,5.3,10.));
#23508=CARTESIAN_POINT('Origin',(6.,-7.6,10.));
#23509=CARTESIAN_POINT('',(4.1,5.,10.));
#23510=CARTESIAN_POINT('Origin',(6.,5.,10.));
#23511=CARTESIAN_POINT('',(4.1,-7.6,10.));
#23512=CARTESIAN_POINT('Origin',(6.,-7.6,10.));
#23513=CARTESIAN_POINT('',(3.65,-5.3,10.));
#23514=CARTESIAN_POINT('',(3.65,-7.6,10.));
#23515=CARTESIAN_POINT('Origin',(6.,-5.3,10.));
#23516=CARTESIAN_POINT('Origin',(6.,-5.3,10.));
#23517=CARTESIAN_POINT('',(4.1,-5.3,10.));
#23518=CARTESIAN_POINT('',(6.25,-5.3,10.));
#23519=CARTESIAN_POINT('Origin',(6.,-5.3,10.));
#23520=CARTESIAN_POINT('Origin',(6.,-7.6,10.));
#23521=CARTESIAN_POINT('',(4.1,-7.6,10.));
#23522=CARTESIAN_POINT('Origin',(6.5,0.,10.));
#23523=CARTESIAN_POINT('',(1.6,-5.5,10.));
#23524=CARTESIAN_POINT('',(1.6,-7.6,10.));
#23525=CARTESIAN_POINT('',(1.2,-5.5,10.));
#23526=CARTESIAN_POINT('',(3.25,-5.5,10.));
#23527=CARTESIAN_POINT('',(1.2,-7.6,10.));
#23528=CARTESIAN_POINT('Origin',(6.5,0.,10.));
#23529=CARTESIAN_POINT('',(1.2,5.,10.));
#23530=CARTESIAN_POINT('',(11.45,5.,10.));
#23531=CARTESIAN_POINT('',(1.2,5.5,10.));
#23532=CARTESIAN_POINT('',(1.2,-7.6,10.));
#23533=CARTESIAN_POINT('',(1.6,5.5,10.));
#23534=CARTESIAN_POINT('',(3.25,5.5,10.));
#23535=CARTESIAN_POINT('',(1.6,5.5,10.));
#23536=CARTESIAN_POINT('Origin',(-1.41421356237309,6.1,11.4142135623731));
#23537=CARTESIAN_POINT('',(-1.57921356237309,6.1,11.4142135623731));
#23538=CARTESIAN_POINT('Origin',(-1.41421356237309,6.1,11.4142135623731));
#23539=CARTESIAN_POINT('',(-1.57921356237309,6.1,11.4142135623731));
#23540=CARTESIAN_POINT('Origin',(-1.41421356237309,6.1,11.4142135623731));
#23541=CARTESIAN_POINT('Origin',(1.4142135623731,6.1,11.4142135623731));
#23542=CARTESIAN_POINT('',(1.2492135623731,6.1,11.4142135623731));
#23543=CARTESIAN_POINT('Origin',(1.4142135623731,6.1,11.4142135623731));
#23544=CARTESIAN_POINT('',(1.2492135623731,6.1,11.4142135623731));
#23545=CARTESIAN_POINT('Origin',(1.4142135623731,6.1,11.4142135623731));
#23546=CARTESIAN_POINT('Origin',(-1.41421356237309,-7.6,11.4142135623731));
#23547=CARTESIAN_POINT('',(-1.57921356237309,-6.1,11.4142135623731));
#23548=CARTESIAN_POINT('',(-1.57921356237309,-7.6,11.4142135623731));
#23549=CARTESIAN_POINT('Origin',(-1.41421356237309,-6.1,11.4142135623731));
#23550=CARTESIAN_POINT('Origin',(-1.41421356237309,-6.1,11.4142135623731));
#23551=CARTESIAN_POINT('Origin',(1.4142135623731,-7.6,11.4142135623731));
#23552=CARTESIAN_POINT('',(1.2492135623731,-6.1,11.4142135623731));
#23553=CARTESIAN_POINT('',(1.2492135623731,-7.6,11.4142135623731));
#23554=CARTESIAN_POINT('Origin',(1.4142135623731,-6.1,11.4142135623731));
#23555=CARTESIAN_POINT('Origin',(1.4142135623731,-6.1,11.4142135623731));
#23556=CARTESIAN_POINT('Origin',(0.,5.5,10.));
#23557=CARTESIAN_POINT('',(-1.6,5.5,10.));
#23558=CARTESIAN_POINT('Origin',(0.,5.5,10.));
#23559=CARTESIAN_POINT('',(-1.6,5.5,10.));
#23560=CARTESIAN_POINT('Origin',(0.,5.5,10.));
#23561=CARTESIAN_POINT('',(-1.2,5.5,10.));
#23562=CARTESIAN_POINT('Origin',(0.,5.5,10.));
#23563=CARTESIAN_POINT('',(3.25,5.5,10.));
#23564=CARTESIAN_POINT('Origin',(0.,-7.6,10.));
#23565=CARTESIAN_POINT('',(-1.6,-5.5,10.));
#23566=CARTESIAN_POINT('',(-1.6,-7.6,10.));
#23567=CARTESIAN_POINT('Origin',(0.,-5.5,10.));
#23568=CARTESIAN_POINT('Origin',(0.,-5.5,10.));
#23569=CARTESIAN_POINT('',(-1.2,-5.5,10.));
#23570=CARTESIAN_POINT('',(3.25,-5.5,10.));
#23571=CARTESIAN_POINT('Origin',(0.,-5.5,10.));
#23572=CARTESIAN_POINT('Origin',(0.,-7.6,10.));
#23573=CARTESIAN_POINT('',(-1.2,-7.6,10.));
#23574=CARTESIAN_POINT('Origin',(0.,-7.6,10.));
#23575=CARTESIAN_POINT('',(-1.2,5.,10.));
#23576=CARTESIAN_POINT('Origin',(0.,5.,10.));
#23577=CARTESIAN_POINT('',(-1.2,-7.6,10.));
#23578=CARTESIAN_POINT('Origin',(16.4,5.,9.9));
#23579=CARTESIAN_POINT('',(16.4,5.,15.));
#23580=CARTESIAN_POINT('',(16.4,5.,9.9));
#23581=CARTESIAN_POINT('',(-3.2,5.,15.));
#23582=CARTESIAN_POINT('',(16.4,5.,15.));
#23583=CARTESIAN_POINT('',(-3.2,5.,10.));
#23584=CARTESIAN_POINT('',(-3.2,5.,9.9));
#23585=CARTESIAN_POINT('',(11.45,5.,10.));
#23586=CARTESIAN_POINT('Origin',(6.5,0.,10.));
#23587=CARTESIAN_POINT('',(-3.2,2.5,10.));
#23588=CARTESIAN_POINT('',(-5.5,7.5,10.));
#23589=CARTESIAN_POINT('',(-4.9,3.,10.));
#23590=CARTESIAN_POINT('Origin',(-4.75,3.,10.));
#23591=CARTESIAN_POINT('',(-5.08,-6.,10.));
#23592=CARTESIAN_POINT('Origin',(-4.75,-6.,10.));
#23593=CARTESIAN_POINT('',(-5.08,-4.04133443718627E-17,10.));
#23594=CARTESIAN_POINT('Origin',(-4.75,0.,10.));
#23595=CARTESIAN_POINT('',(-5.08,6.,10.));
#23596=CARTESIAN_POINT('Origin',(-4.75,6.,10.));
#23597=CARTESIAN_POINT('',(-4.9,-3.,10.));
#23598=CARTESIAN_POINT('Origin',(-4.75,-3.,10.));
#23599=CARTESIAN_POINT('Origin',(17.75,3.,9.5));
#23600=CARTESIAN_POINT('',(17.6,3.,10.5));
#23601=CARTESIAN_POINT('',(17.6,3.,9.5));
#23602=CARTESIAN_POINT('Origin',(17.75,3.,10.5));
#23603=CARTESIAN_POINT('Origin',(17.75,3.,10.5));
#23604=CARTESIAN_POINT('Origin',(17.75,-3.,9.5));
#23605=CARTESIAN_POINT('',(17.6,-3.,10.5));
#23606=CARTESIAN_POINT('',(17.6,-3.,9.5));
#23607=CARTESIAN_POINT('Origin',(17.75,-3.,10.5));
#23608=CARTESIAN_POINT('Origin',(17.75,-3.,10.5));
#23609=CARTESIAN_POINT('Origin',(-4.75,3.,9.5));
#23610=CARTESIAN_POINT('',(-4.9,3.,10.5));
#23611=CARTESIAN_POINT('',(-4.9,3.,9.5));
#23612=CARTESIAN_POINT('Origin',(-4.75,3.,10.5));
#23613=CARTESIAN_POINT('Origin',(-4.75,3.,10.5));
#23614=CARTESIAN_POINT('Origin',(-4.75,-3.,9.5));
#23615=CARTESIAN_POINT('',(-4.9,-3.,10.5));
#23616=CARTESIAN_POINT('',(-4.9,-3.,9.5));
#23617=CARTESIAN_POINT('Origin',(-4.75,-3.,10.5));
#23618=CARTESIAN_POINT('Origin',(-4.75,-3.,10.5));
#23619=CARTESIAN_POINT('Origin',(17.75,0.,9.9));
#23620=CARTESIAN_POINT('',(17.42,4.04133443718624E-17,10.8));
#23621=CARTESIAN_POINT('',(17.42,-4.04133443718624E-17,9.9));
#23622=CARTESIAN_POINT('Origin',(17.75,0.,10.8));
#23623=CARTESIAN_POINT('Origin',(-4.75,-6.,9.9));
#23624=CARTESIAN_POINT('',(-5.08,-6.,10.8));
#23625=CARTESIAN_POINT('',(-5.08,-6.,9.9));
#23626=CARTESIAN_POINT('Origin',(-4.75,-6.,10.8));
#23627=CARTESIAN_POINT('Origin',(-4.75,0.,9.9));
#23628=CARTESIAN_POINT('',(-5.08,4.04133443718627E-17,10.8));
#23629=CARTESIAN_POINT('',(-5.08,-4.04133443718627E-17,9.9));
#23630=CARTESIAN_POINT('Origin',(-4.75,0.,10.8));
#23631=CARTESIAN_POINT('Origin',(-4.75,6.,9.9));
#23632=CARTESIAN_POINT('',(-5.08,6.,10.8));
#23633=CARTESIAN_POINT('',(-5.08,6.,9.9));
#23634=CARTESIAN_POINT('Origin',(-4.75,6.,10.8));
#23635=CARTESIAN_POINT('Origin',(17.75,-6.,9.9));
#23636=CARTESIAN_POINT('',(17.42,-6.,10.8));
#23637=CARTESIAN_POINT('',(17.42,-6.,9.9));
#23638=CARTESIAN_POINT('Origin',(17.75,-6.,10.8));
#23639=CARTESIAN_POINT('Origin',(17.75,6.,9.9));
#23640=CARTESIAN_POINT('',(17.42,6.,10.8));
#23641=CARTESIAN_POINT('',(17.42,6.,9.9));
#23642=CARTESIAN_POINT('Origin',(17.75,6.,10.8));
#23643=CARTESIAN_POINT('Origin',(18.5,-7.5,10.));
#23644=CARTESIAN_POINT('',(18.5,-7.5,10.8));
#23645=CARTESIAN_POINT('Origin',(17.75,0.,10.8));
#23646=CARTESIAN_POINT('',(17.,-3.75,10.8));
#23647=CARTESIAN_POINT('Origin',(-5.5,7.5,10.));
#23648=CARTESIAN_POINT('',(-5.5,7.5,10.8));
#23649=CARTESIAN_POINT('Origin',(-4.75,0.,10.8));
#23650=CARTESIAN_POINT('',(-4.,3.75,10.8));
#23651=CARTESIAN_POINT('Origin',(-4.,7.5,10.));
#23652=CARTESIAN_POINT('',(-4.,7.5,16.));
#23653=CARTESIAN_POINT('Origin',(16.4,-5.,9.9));
#23654=CARTESIAN_POINT('',(16.4,-5.,15.));
#23655=CARTESIAN_POINT('Origin',(-3.2,5.,9.9));
#23656=CARTESIAN_POINT('',(-3.2,5.,15.));
#23657=CARTESIAN_POINT('Origin',(6.6,0.,15.));
#23658=CARTESIAN_POINT('Origin',(17.,-7.5,10.));
#23659=CARTESIAN_POINT('',(17.,-7.5,16.));
#23660=CARTESIAN_POINT('Origin',(6.5,0.,16.));
#73243=UNCERTAINTY_MEASURE_WITH_UNIT(LENGTH_MEASURE(0.001),#73367,
'DISTANCE_ACCURACY_VALUE',
'Maximum model space distance between geometric entities at asserted c
onnectivities');
#73302=UNCERTAINTY_MEASURE_WITH_UNIT(LENGTH_MEASURE(0.001),#73367,
'DISTANCE_ACCURACY_VALUE',
'Maximum model space distance between geometric entities at asserted c
onnectivities');
#73307=(
GEOMETRIC_REPRESENTATION_CONTEXT(3)
GLOBAL_UNCERTAINTY_ASSIGNED_CONTEXT((#73243))
GLOBAL_UNIT_ASSIGNED_CONTEXT((#73367,#73369,#73370))
REPRESENTATION_CONTEXT('','3D')
);
#73366=(
GEOMETRIC_REPRESENTATION_CONTEXT(3)
GLOBAL_UNCERTAINTY_ASSIGNED_CONTEXT((#73302))
GLOBAL_UNIT_ASSIGNED_CONTEXT((#73367,#73369,#73370))
REPRESENTATION_CONTEXT('','3D')
);
#73367=(
LENGTH_UNIT()
NAMED_UNIT(*)
SI_UNIT(.CENTI.,.METRE.)
);
#73369=(
NAMED_UNIT(*)
PLANE_ANGLE_UNIT()
SI_UNIT($,.RADIAN.)
);
#73370=(
NAMED_UNIT(*)
SI_UNIT($,.STERADIAN.)
SOLID_ANGLE_UNIT()
);
#73375=SHAPE_DEFINITION_REPRESENTATION(#73438,#73611);
#73438=PRODUCT_DEFINITION_SHAPE('',$,#73675);
#73611=SHAPE_REPRESENTATION('',(#17006),#73307);
#73670=PRODUCT_DEFINITION_CONTEXT('part definition',#73861,'design');
#73675=PRODUCT_DEFINITION('Upper housing','Upper housing',#73738,#73670);
#73738=PRODUCT_DEFINITION_FORMATION('',$,#73867);
#73861=APPLICATION_CONTEXT(
'Core Data for Automotive Mechanical Design Process');
#73862=PRODUCT_CONTEXT('part definition',#73861,'mechanical');
#73867=PRODUCT('Upper housing','Upper housing','Upper housing',(#73862));
#73961=COLOUR_RGB('Dark Blue',0.08,0.2,0.34);
#73962=FILL_AREA_STYLE_COLOUR('',#73961);
#73963=FILL_AREA_STYLE('',(#73962));
#73964=SURFACE_STYLE_FILL_AREA(#73963);
#73965=SURFACE_SIDE_STYLE('',(#73964));
#73966=SURFACE_STYLE_USAGE(.BOTH.,#73965);
#73967=PRESENTATION_STYLE_ASSIGNMENT((#73966));
ENDSEC;
END-ISO-10303-21;
